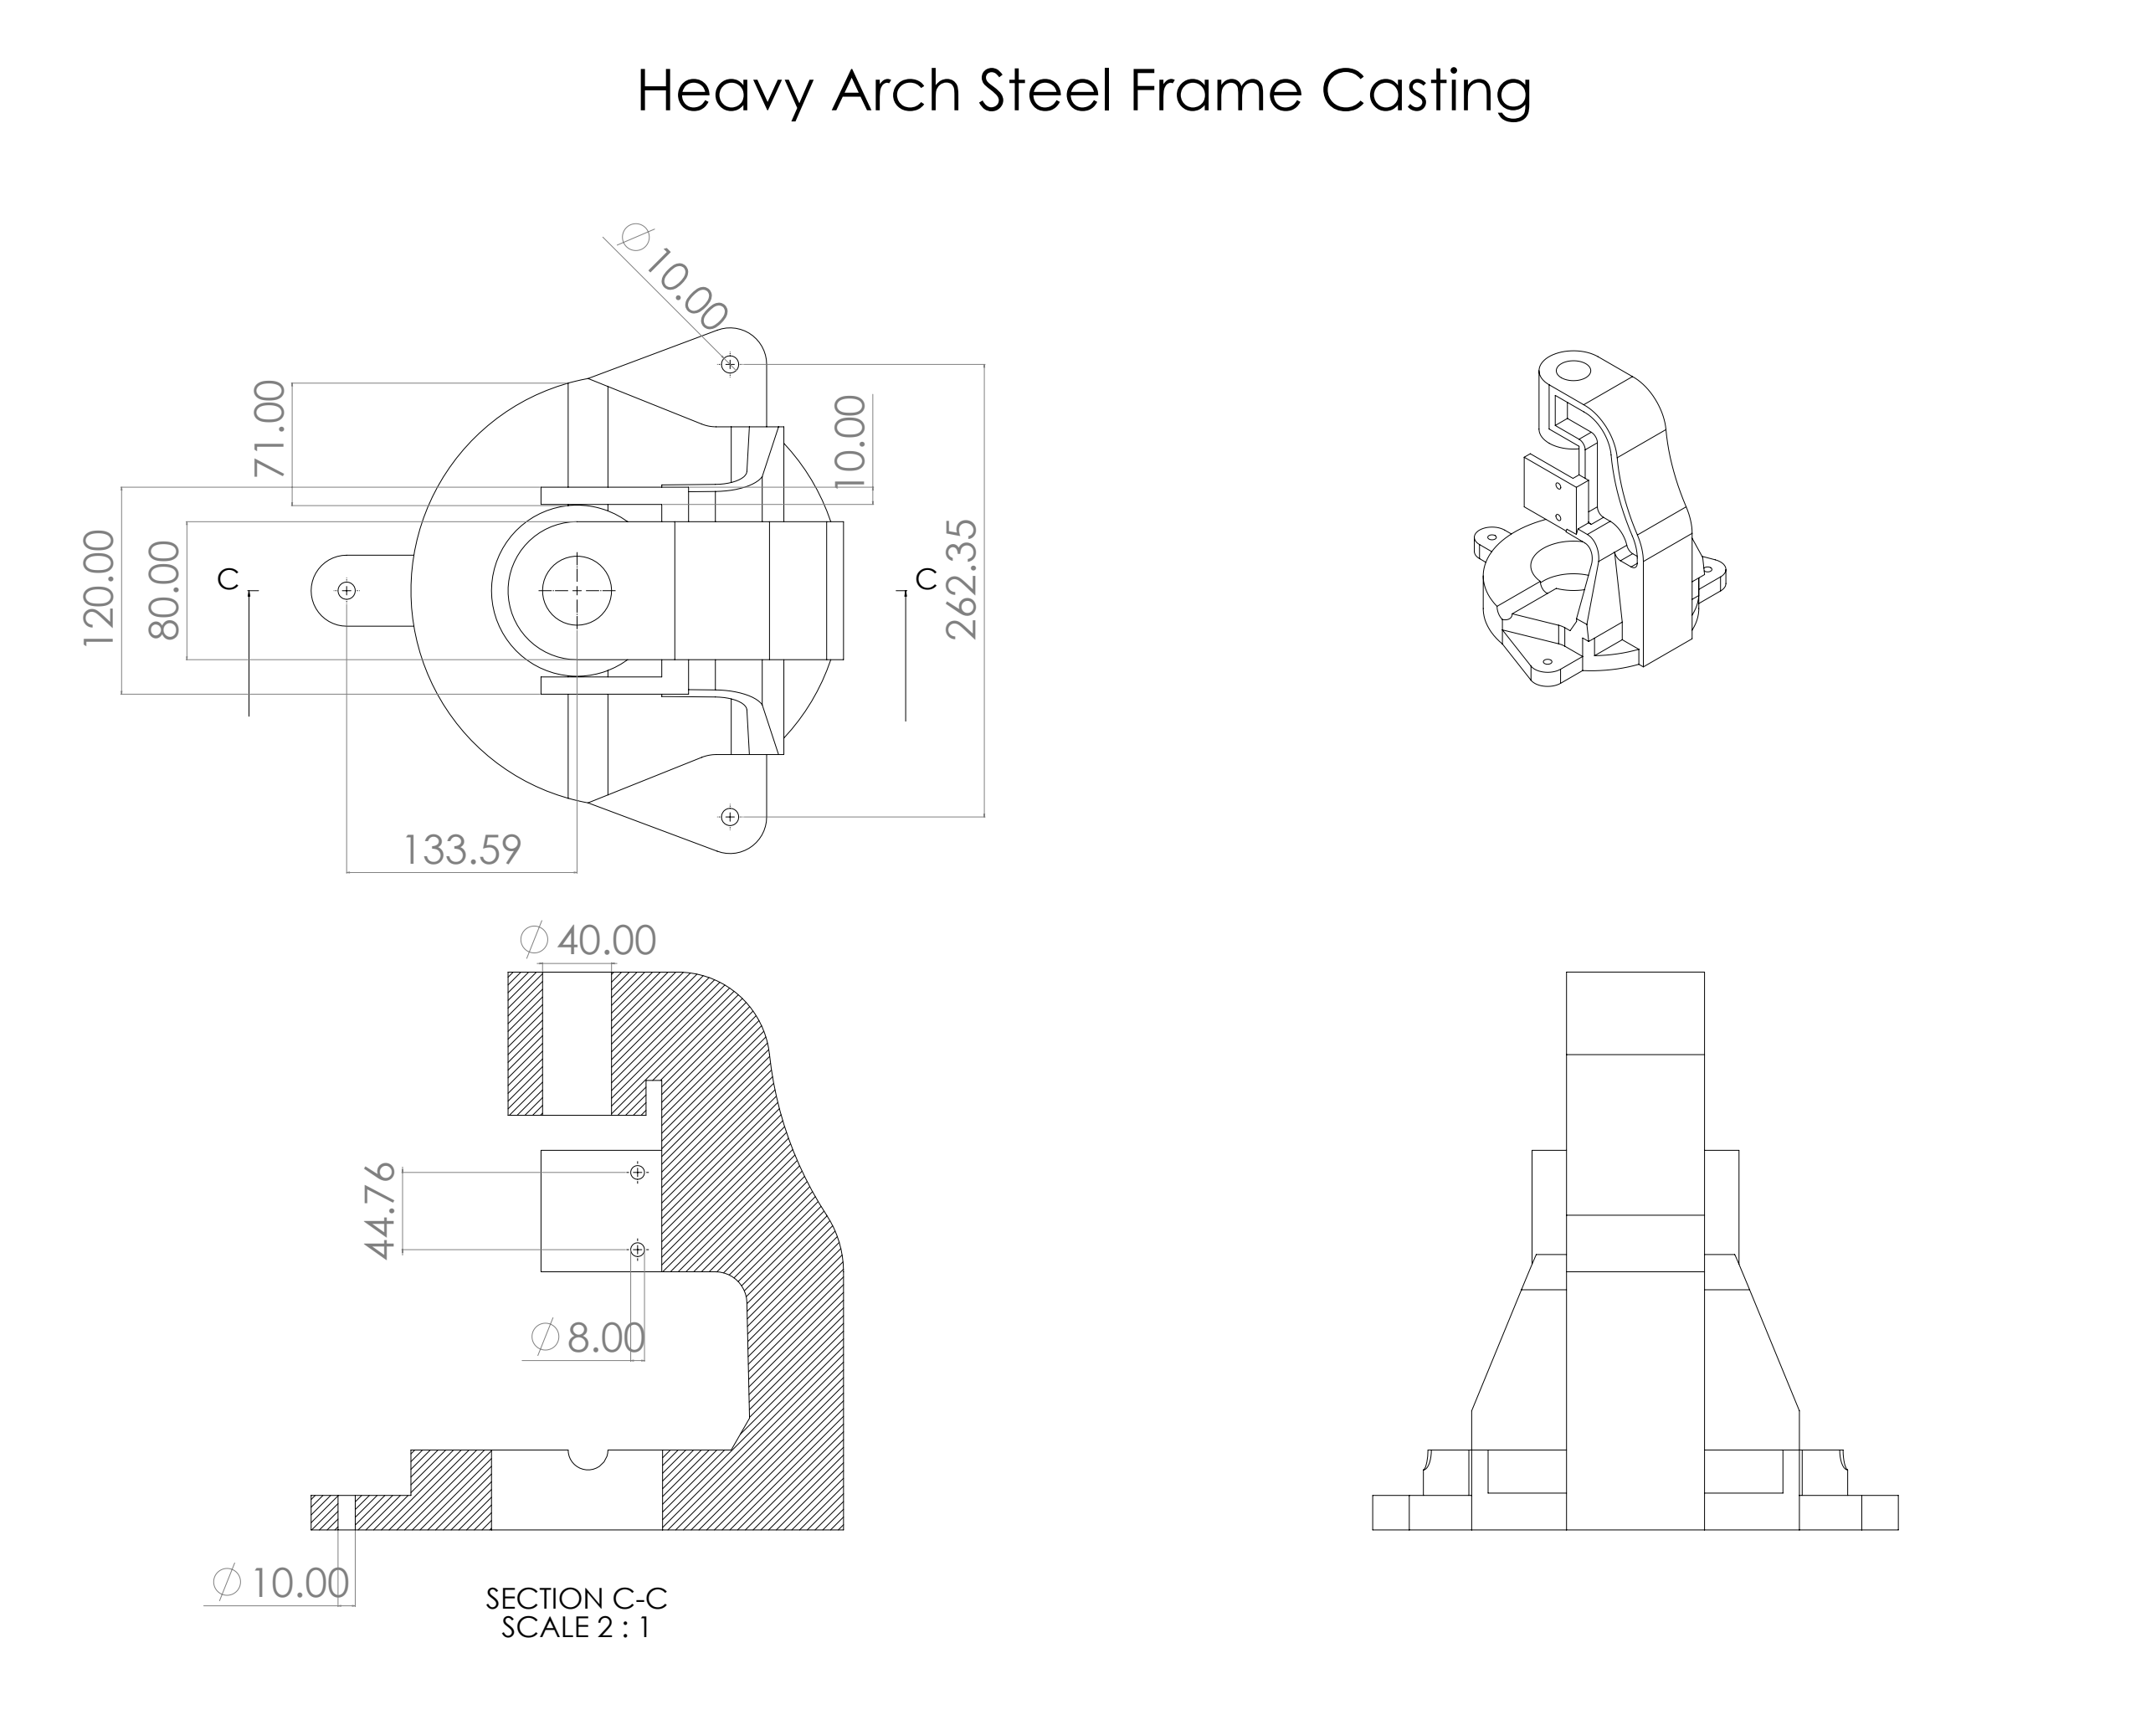
ISO-10303-21;
HEADER;
FILE_DESCRIPTION (('STEP AP214'),
    '1' );
FILE_NAME ('Heavy Arch Steel Frame Casting.step',
    '2026-10-24T00:28:05',
    ( '' ),
    ( '' ),
    'SwSTEP 2.0',
    'SolidWorks 2025',
    '' );
FILE_SCHEMA (( 'AUTOMOTIVE_DESIGN' ));
ENDSEC;

DATA;
#3=VECTOR ( 'NONE', #11444, 1000.000000000000000 ) ;
#4=DIRECTION ( 'NONE',  ( 0.000000000000000000, -1.000000000000000000, 0.000000000000000000 ) ) ;
#8=DIRECTION ( 'NONE',  ( -0.000000000000000000, -0.000000000000000000, -1.000000000000000000 ) ) ;
#9=ORIENTED_EDGE ( 'NONE', *, *, #63, .F. ) ;
#13=VERTEX_POINT ( 'NONE', #14894 ) ;
#23=CARTESIAN_POINT ( 'NONE',  ( 20.42502041961814641, 160.1716627696692683, -50.00000000000000000 ) ) ;
#25=DIRECTION ( 'NONE',  ( 0.000000000000000000, 0.000000000000000000, 1.000000000000000000 ) ) ;
#26=AXIS2_PLACEMENT_3D ( 'NONE', #1810, #8485, #15108 ) ;
#28=CARTESIAN_POINT ( 'NONE',  ( -33.09803238365465461, 52.74628974220605215, 120.5385558893279807 ) ) ;
#30=CARTESIAN_POINT ( 'NONE',  ( -10.76731745429009912, 56.85652257517428865, 118.3724535612433186 ) ) ;
#32=( GEOMETRIC_REPRESENTATION_CONTEXT ( 3 ) GLOBAL_UNCERTAINTY_ASSIGNED_CONTEXT ( ( #4204 ) ) GLOBAL_UNIT_ASSIGNED_CONTEXT ( ( #10723, #14002, #17024 ) ) REPRESENTATION_CONTEXT ( 'NONE', 'WORKASPACE' ) );
#35=ORIENTED_EDGE ( 'NONE', *, *, #14468, .F. ) ;
#40=AXIS2_PLACEMENT_3D ( 'NONE', #19318, #13155, #16192 ) ;
#59=CARTESIAN_POINT ( 'NONE',  ( 115.7989814974898337, 152.5259582928263740, 40.00000000000000000 ) ) ;
#60=DIRECTION ( 'NONE',  ( 1.000000000000000000, 9.855701800883827197E-17, 0.000000000000000000 ) ) ;
#63=EDGE_CURVE ( 'NONE', #14197, #16401, #15913, .T. ) ;
#68=CARTESIAN_POINT ( 'NONE',  ( -22.30770786884145451, -343.0245277843623057, -122.9933582338429687 ) ) ;
#70=CARTESIAN_POINT ( 'NONE',  ( 20.42502041961814641, 160.1716627696692683, 49.99999999999999289 ) ) ;
#73=ADVANCED_FACE ( 'NONE', ( #292 ), #3940, .T. ) ;
#85=CARTESIAN_POINT ( 'NONE',  ( -11.33174043645153262, 53.25345476394927857, -46.46619372074344767 ) ) ;
#89=FACE_OUTER_BOUND ( 'NONE', #5371, .T. ) ;
#91=DIRECTION ( 'NONE',  ( 1.854788578061058554E-16, 1.000000000000000000, 0.000000000000000000 ) ) ;
#94=CARTESIAN_POINT ( 'NONE',  ( -10.76731745429010090, 56.85652257517428865, -152.3753892284480003 ) ) ;
#96=DIRECTION ( 'NONE',  ( -1.000000000000000000, 0.000000000000000000, 0.000000000000000000 ) ) ;
#100=CARTESIAN_POINT ( 'NONE',  ( -28.68588794268872277, 230.8848358243226073, -40.00000000000000000 ) ) ;
#105=ORIENTED_EDGE ( 'NONE', *, *, #199, .F. ) ;
#107=EDGE_CURVE ( 'NONE', #16081, #2296, #14541, .T. ) ;
#113=EDGE_CURVE ( 'NONE', #8154, #14441, #20281, .T. ) ;
#116=CARTESIAN_POINT ( 'NONE',  ( 69.79185940953689737, 142.2976266388001250, 69.11456258820065557 ) ) ;
#117=AXIS2_PLACEMENT_3D ( 'NONE', #15282, #17003, #20238 ) ;
#123=ORIENTED_EDGE ( 'NONE', *, *, #2940, .T. ) ;
#132=ORIENTED_EDGE ( 'NONE', *, *, #11871, .F. ) ;
#146=CARTESIAN_POINT ( 'NONE',  ( 20.42502041961814641, 160.1716627696692683, 61.32762281133329196 ) ) ;
#150=VECTOR ( 'NONE', #6440, 1000.000000000000000 ) ;
#154=VECTOR ( 'NONE', #10153, 1000.000000000000000 ) ;
#155=ORIENTED_EDGE ( 'NONE', *, *, #15237, .F. ) ;
#157=EDGE_LOOP ( 'NONE', ( #5136, #14998, #4320, #2465 ) ) ;
#168=DIRECTION ( 'NONE',  ( 0.000000000000000000, 0.000000000000000000, -1.000000000000000000 ) ) ;
#174=LINE ( 'NONE', #10093, #7830 ) ;
#179=EDGE_CURVE ( 'NONE', #20702, #11681, #8806, .T. ) ;
#182=VERTEX_POINT ( 'NONE', #608 ) ;
#184=ORIENTED_EDGE ( 'NONE', *, *, #5125, .F. ) ;
#188=ORIENTED_EDGE ( 'NONE', *, *, #12536, .T. ) ;
#193=CARTESIAN_POINT ( 'NONE',  ( -18.46114582419561856, 45.97303840584705625, -48.53623208051946136 ) ) ;
#195=CARTESIAN_POINT ( 'NONE',  ( 71.32175588950862277, 75.31183677523708297, 40.00000000000000000 ) ) ;
#199=EDGE_CURVE ( 'NONE', #182, #19453, #6902, .T. ) ;
#206=CARTESIAN_POINT ( 'NONE',  ( -31.47597222270714212, 49.78415940255306538, -49.52648848774079937 ) ) ;
#216=ORIENTED_EDGE ( 'NONE', *, *, #18810, .T. ) ;
#219=EDGE_CURVE ( 'NONE', #12803, #14751, #2645, .T. ) ;
#227=CARTESIAN_POINT ( 'NONE',  ( 60.03793209889851568, 30.52886280891152282, -131.1729372809869005 ) ) ;
#230=ORIENTED_EDGE ( 'NONE', *, *, #2551, .F. ) ;
#234=ORIENTED_EDGE ( 'NONE', *, *, #8898, .F. ) ;
#243=VECTOR ( 'NONE', #20484, 1000.000000000000000 ) ;
#245=DIRECTION ( 'NONE',  ( -1.000000000000000000, 0.000000000000000000, 0.000000000000000000 ) ) ;
#258=VERTEX_POINT ( 'NONE', #20385 ) ;
#264=VERTEX_POINT ( 'NONE', #824 ) ;
#281=CARTESIAN_POINT ( 'NONE',  ( 79.78925230247502043, 142.5259582928263455, -20.00000000000000355 ) ) ;
#292=FACE_OUTER_BOUND ( 'NONE', #157, .T. ) ;
#297=CARTESIAN_POINT ( 'NONE',  ( -13.97728958318061565, 48.85369832438319548, -47.37148056848186428 ) ) ;
#299=DIRECTION ( 'NONE',  ( 1.000000000000000000, 0.000000000000000000, 0.000000000000000000 ) ) ;
#300=EDGE_CURVE ( 'NONE', #14946, #18462, #14017, .T. ) ;
#305=DIRECTION ( 'NONE',  ( 0.000000000000000000, 1.000000000000000000, 0.000000000000000000 ) ) ;
#310=CARTESIAN_POINT ( 'NONE',  ( -28.68588794268872988, 47.23886018424757083, -49.60091809715359545 ) ) ;
#317=ORIENTED_EDGE ( 'NONE', *, *, #11658, .T. ) ;
#323=AXIS2_PLACEMENT_3D ( 'NONE', #6998, #18893, #7103 ) ;
#352=VECTOR ( 'NONE', #18176, 1000.000000000000000 ) ;
#359=CARTESIAN_POINT ( 'NONE',  ( 0.000000000000000000, 56.85652257517428865, 0.000000000000000000 ) ) ;
#376=VECTOR ( 'NONE', #7717, 1000.000000000000000 ) ;
#385=CARTESIAN_POINT ( 'NONE',  ( 30.42502041961813575, 271.1055109169419097, 20.00000000000000355 ) ) ;
#387=CARTESIAN_POINT ( 'NONE',  ( 81.24038404635966515, 10.52886280891152104, -94.99999999999994316 ) ) ;
#389=ADVANCED_FACE ( 'NONE', ( #7915 ), #13016, .F. ) ;
#392=CIRCLE ( 'NONE', #11415, 9.999999999999994671 ) ;
#393=CARTESIAN_POINT ( 'NONE',  ( 81.24038404635966515, 10.52886280891152104, 94.99999999999994316 ) ) ;
#396=ORIENTED_EDGE ( 'NONE', *, *, #3873, .T. ) ;
#399=VECTOR ( 'NONE', #1589, 1000.000000000000000 ) ;
#402=EDGE_LOOP ( 'NONE', ( #20811, #2569, #4602, #6698 ) ) ;
#407=CARTESIAN_POINT ( 'NONE',  ( -28.68588794268872988, 47.23886018424757083, -49.60091809715359545 ) ) ;
#411=DIRECTION ( 'NONE',  ( 0.000000000000000000, -1.000000000000000000, 0.000000000000000000 ) ) ;
#426=ORIENTED_EDGE ( 'NONE', *, *, #17683, .T. ) ;
#428=CARTESIAN_POINT ( 'NONE',  ( 30.07572094023280940, 170.1716627696692683, -57.31989048965873934 ) ) ;
#430=ORIENTED_EDGE ( 'NONE', *, *, #1923, .F. ) ;
#431=FACE_OUTER_BOUND ( 'NONE', #16031, .T. ) ;
#440=EDGE_CURVE ( 'NONE', #16030, #15607, #16966, .T. ) ;
#443=ORIENTED_EDGE ( 'NONE', *, *, #8517, .T. ) ;
#446=ORIENTED_EDGE ( 'NONE', *, *, #9956, .F. ) ;
#450=AXIS2_PLACEMENT_3D ( 'NONE', #15921, #17640, #8987 ) ;
#451=VERTEX_POINT ( 'NONE', #3287 ) ;
#454=VERTEX_POINT ( 'NONE', #16805 ) ;
#464=CARTESIAN_POINT ( 'NONE',  ( -26.01014438536011397, 45.91972051657856468, 122.2644972899424687 ) ) ;
#466=LINE ( 'NONE', #566, #15334 ) ;
#475=ORIENTED_EDGE ( 'NONE', *, *, #15442, .F. ) ;
#493=AXIS2_PLACEMENT_3D ( 'NONE', #1831, #8402, #15027 ) ;
#494=CARTESIAN_POINT ( 'NONE',  ( 81.24038404635965094, 10.52886280891152104, -131.1729372809869005 ) ) ;
#496=AXIS2_PLACEMENT_3D ( 'NONE', #18707, #14078, #15484 ) ;
#504=EDGE_LOOP ( 'NONE', ( #18852, #5687, #1345, #9828 ) ) ;
#509=ORIENTED_EDGE ( 'NONE', *, *, #7343, .F. ) ;
#514=CARTESIAN_POINT ( 'NONE',  ( 52.60622592008805043, 30.52886280891152282, -151.0302712373927250 ) ) ;
#525=DIRECTION ( 'NONE',  ( -0.000000000000000000, -0.000000000000000000, -1.000000000000000000 ) ) ;
#527=ORIENTED_EDGE ( 'NONE', *, *, #5440, .F. ) ;
#534=VERTEX_POINT ( 'NONE', #5742 ) ;
#549=ORIENTED_EDGE ( 'NONE', *, *, #4990, .T. ) ;
#554=VERTEX_POINT ( 'NONE', #14098 ) ;
#566=CARTESIAN_POINT ( 'NONE',  ( -74.06037022053952512, 10.52886280891152104, -40.00000000000000000 ) ) ;
#572=EDGE_LOOP ( 'NONE', ( #20946, #19765, #20650 ) ) ;
#588=CARTESIAN_POINT ( 'NONE',  ( 35.96497763894178945, 230.5765313837437418, -40.00000000000000000 ) ) ;
#592=DIRECTION ( 'NONE',  ( -0.000000000000000000, -0.000000000000000000, -1.000000000000000000 ) ) ;
#595=EDGE_CURVE ( 'NONE', #1881, #15561, #10610, .T. ) ;
#596=CIRCLE ( 'NONE', #11637, 4.000000000000003553 ) ;
#602=ORIENTED_EDGE ( 'NONE', *, *, #17756, .T. ) ;
#604=VERTEX_POINT ( 'NONE', #20679 ) ;
#606=LINE ( 'NONE', #100, #18425 ) ;
#607=EDGE_CURVE ( 'NONE', #10104, #12829, #18832, .T. ) ;
#608=CARTESIAN_POINT ( 'NONE',  ( -28.68588794268874054, 271.1055109169419666, 40.00000000000000000 ) ) ;
#610=ORIENTED_EDGE ( 'NONE', *, *, #4427, .T. ) ;
#615=LINE ( 'NONE', #17154, #5483 ) ;
#632=ORIENTED_EDGE ( 'NONE', *, *, #5260, .T. ) ;
#639=CARTESIAN_POINT ( 'NONE',  ( -28.68588794268873698, 10.52886280891152104, 0.000000000000000000 ) ) ;
#647=CARTESIAN_POINT ( 'NONE',  ( 60.03793209889851568, 30.52886280891152282, 131.1729372809869005 ) ) ;
#649=ADVANCED_FACE ( 'NONE', ( #4241 ), #12780, .T. ) ;
#651=DIRECTION ( 'NONE',  ( -0.000000000000000000, -0.000000000000000000, 1.000000000000000000 ) ) ;
#653=CIRCLE ( 'NONE', #14480, 21.20245194746113526 ) ;
#671=AXIS2_PLACEMENT_3D ( 'NONE', #5649, #6070, #7583 ) ;
#680=EDGE_LOOP ( 'NONE', ( #16620, #509, #5345, #8208 ) ) ;
#684=CARTESIAN_POINT ( 'NONE',  ( 115.7989814974898337, 152.5259582928263740, -20.00000000000000355 ) ) ;
#696=DIRECTION ( 'NONE',  ( 1.000000000000000000, 0.000000000000000000, 0.000000000000000000 ) ) ;
#698=FACE_OUTER_BOUND ( 'NONE', #4314, .T. ) ;
#700=DIRECTION ( 'NONE',  ( -0.000000000000000000, -0.000000000000000000, -1.000000000000000000 ) ) ;
#703=DIRECTION ( 'NONE',  ( 0.000000000000000000, -1.000000000000000000, 0.000000000000000000 ) ) ;
#706=ORIENTED_EDGE ( 'NONE', *, *, #13101, .F. ) ;
#714=ORIENTED_EDGE ( 'NONE', *, *, #20644, .F. ) ;
#717=EDGE_CURVE ( 'NONE', #20672, #5108, #13166, .T. ) ;
#723=DIRECTION ( 'NONE',  ( 0.000000000000000000, -0.000000000000000000, -1.000000000000000000 ) ) ;
#727=FACE_OUTER_BOUND ( 'NONE', #18825, .T. ) ;
#728=CLOSED_SHELL ( 'NONE', ( #4202, #18729, #7183, #1313, #6098, #14803, #2877, #2308, #8698, #9259, #1514, #21123, #2681, #8425, #4950, #3532, #389, #2715, #19260, #14653, #15130, #14125, #19463, #13734, #19883, #19785, #7149, #16387, #12129, #10656, #9205, #12272, #16233, #3470, #2143, #15969, #3158, #11966, #8090, #20749, #11190, #649, #18699, #8016, #5574, #907, #20543, #1966, #6567, #13747, #21117, #1097, #12190, #73, #11691, #16866, #10538, #19874, #8200, #12587, #9693, #14131, #2231, #11601, #7880, #15316, #13856, #1907, #10138, #3997, #11879, #20146, #15364, #1047, #17279, #12993, #4417, #13206, #9791, #6710, #19859, #8106, #17682, #4283, #12076, #13479, #20733, #20323, #20863, #3939, #1701, #7829, #2906, #15283, #6218, #20450, #19796, #1639, #4404, #10989, #20740, #14224, #2354, #839, #7752, #14892, #15777, #1840, #3193, #15792, #9164, #1436, #7801, #12477, #8633, #18193, #14455, #9085, #11057 ) ) ;
#730=EDGE_CURVE ( 'NONE', #15685, #3984, #3339, .T. ) ;
#739=VERTEX_POINT ( 'NONE', #17751 ) ;
#754=CARTESIAN_POINT ( 'NONE',  ( 52.94681837068318941, 78.74778544605769071, -94.99999999999994316 ) ) ;
#763=VERTEX_POINT ( 'NONE', #10929 ) ;
#764=CARTESIAN_POINT ( 'NONE',  ( 292.4526463419396691, 308.2087638784415162, 20.00000000000000355 ) ) ;
#765=ORIENTED_EDGE ( 'NONE', *, *, #15458, .T. ) ;
#772=ORIENTED_EDGE ( 'NONE', *, *, #7755, .F. ) ;
#779=DIRECTION ( 'NONE',  ( 0.000000000000000000, -1.000000000000000000, 0.000000000000000000 ) ) ;
#785=PRODUCT_DEFINITION_CONTEXT ( 'detailed design', #9294, 'design' ) ;
#790=AXIS2_PLACEMENT_3D ( 'NONE', #4343, #10924, #17535 ) ;
#793=ORIENTED_EDGE ( 'NONE', *, *, #1569, .T. ) ;
#795=VERTEX_POINT ( 'NONE', #9310 ) ;
#796=LINE ( 'NONE', #2405, #6289 ) ;
#806=DIRECTION ( 'NONE',  ( -0.000000000000000000, -0.000000000000000000, 1.000000000000000000 ) ) ;
#808=CARTESIAN_POINT ( 'NONE',  ( 0.000000000000000000, 0.000000000000000000, 0.000000000000000000 ) ) ;
#814=CARTESIAN_POINT ( 'NONE',  ( -33.24036626417445461, 53.08430543508956134, -120.4996691248974656 ) ) ;
#824=CARTESIAN_POINT ( 'NONE',  ( -49.57497958038186425, 230.5765313837437418, 60.00000000000000000 ) ) ;
#834=DIRECTION ( 'NONE',  ( 1.000000000000000000, 0.000000000000000000, 0.000000000000000000 ) ) ;
#835=CARTESIAN_POINT ( 'NONE',  ( 6.416697501590670427, 172.9933428177121471, -60.00000000000000000 ) ) ;
#836=CIRCLE ( 'NONE', #10824, 21.20245194746113526 ) ;
#839=ADVANCED_FACE ( 'NONE', ( #6238 ), #6566, .T. ) ;
#840=CARTESIAN_POINT ( 'NONE',  ( 6.416697501590670427, 217.7548513357008630, 49.99999999999999289 ) ) ;
#847=ORIENTED_EDGE ( 'NONE', *, *, #2670, .F. ) ;
#851=CARTESIAN_POINT ( 'NONE',  ( 105.7989814974898479, 152.5259582928263740, 20.00000000000000355 ) ) ;
#857=FACE_OUTER_BOUND ( 'NONE', #9920, .T. ) ;
#858=CARTESIAN_POINT ( 'NONE',  ( -28.68588794268872277, 174.3162933293988033, -20.00000000000000000 ) ) ;
#861=DIRECTION ( 'NONE',  ( 0.000000000000000000, -1.000000000000000000, 0.000000000000000000 ) ) ;
#865=DIRECTION ( 'NONE',  ( -0.000000000000000000, -0.000000000000000000, -1.000000000000000000 ) ) ;
#871=ORIENTED_EDGE ( 'NONE', *, *, #21201, .F. ) ;
#874=EDGE_LOOP ( 'NONE', ( #5710, #13740, #20222, #9194 ) ) ;
#880=VERTEX_POINT ( 'NONE', #1839 ) ;
#889=LINE ( 'NONE', #9296, #7146 ) ;
#895=ORIENTED_EDGE ( 'NONE', *, *, #3138, .F. ) ;
#898=ORIENTED_EDGE ( 'NONE', *, *, #6988, .F. ) ;
#907=ADVANCED_FACE ( 'NONE', ( #11663 ), #10238, .F. ) ;
#912=DIRECTION ( 'NONE',  ( -0.02112707654195870172, 0.9250389998264586522, -0.3792841882241536067 ) ) ;
#928=DIRECTION ( 'NONE',  ( 0.000000000000000000, -1.000000000000000000, 0.000000000000000000 ) ) ;
#931=CYLINDRICAL_SURFACE ( 'NONE', #21088, 125.0000000000000000 ) ;
#939=CARTESIAN_POINT ( 'NONE',  ( 79.78925230247502043, 142.5259582928263455, -40.00000000000000000 ) ) ;
#940=CARTESIAN_POINT ( 'NONE',  ( 20.42502041961813930, 230.5765313837437418, 60.00000000000000000 ) ) ;
#947=VECTOR ( 'NONE', #1680, 1000.000000000000114 ) ;
#948=DIRECTION ( 'NONE',  ( 0.000000000000000000, -1.000000000000000000, 0.000000000000000000 ) ) ;
#950=DIRECTION ( 'NONE',  ( 0.000000000000000000, -1.000000000000000000, 0.000000000000000000 ) ) ;
#952=VERTEX_POINT ( 'NONE', #10343 ) ;
#954=ORIENTED_EDGE ( 'NONE', *, *, #14883, .F. ) ;
#956=AXIS2_PLACEMENT_3D ( 'NONE', #2213, #8797, #5337 ) ;
#961=EDGE_LOOP ( 'NONE', ( #6161, #9124, #13988, #14252 ) ) ;
#970=DIRECTION ( 'NONE',  ( 0.000000000000000000, -1.000000000000000000, 0.000000000000000000 ) ) ;
#973=AXIS2_PLACEMENT_3D ( 'NONE', #2028, #2337, #11954 ) ;
#983=VERTEX_POINT ( 'NONE', #16655 ) ;
#989=ORIENTED_EDGE ( 'NONE', *, *, #1574, .T. ) ;
#997=CARTESIAN_POINT ( 'NONE',  ( 28.16023193154655502, 323.8848358243226357, 40.00000000000000000 ) ) ;
#998=DIRECTION ( 'NONE',  ( -1.374938938973709817E-16, 1.000000000000000000, 0.000000000000000000 ) ) ;
#1002=VERTEX_POINT ( 'NONE', #8832 ) ;
#1007=ORIENTED_EDGE ( 'NONE', *, *, #9742, .T. ) ;
#1017=AXIS2_PLACEMENT_3D ( 'NONE', #12084, #13620, #8731 ) ;
#1019=DIRECTION ( 'NONE',  ( 1.000000000000000000, 0.000000000000000000, 0.000000000000000000 ) ) ;
#1022=CARTESIAN_POINT ( 'NONE',  ( -18.68588794268873698, 323.8848358243226357, -40.00000000000000000 ) ) ;
#1030=ORIENTED_EDGE ( 'NONE', *, *, #13546, .T. ) ;
#1032=EDGE_LOOP ( 'NONE', ( #18693, #12072, #7439, #4372, #20196, #8855, #4075 ) ) ;
#1033=CARTESIAN_POINT ( 'NONE',  ( 115.7989814974898337, 142.5259582928263455, 20.00000000000000355 ) ) ;
#1038=ORIENTED_EDGE ( 'NONE', *, *, #21391, .T. ) ;
#1040=CARTESIAN_POINT ( 'NONE',  ( 72.94945500224395118, 285.0140030772282103, -20.00000000000000355 ) ) ;
#1046=PLANE ( 'NONE',  #18730 ) ;
#1047=ADVANCED_FACE ( 'NONE', ( #431 ), #16968, .F. ) ;
#1049=CIRCLE ( 'NONE', #11375, 210.7252770684331438 ) ;
#1051=CARTESIAN_POINT ( 'NONE',  ( 51.93385628276429600, 30.52886280891152282, 94.99999999999994316 ) ) ;
#1055=CARTESIAN_POINT ( 'NONE',  ( 78.68120802659203150, 149.7457237375499517, 40.00000000000000000 ) ) ;
#1066=ORIENTED_EDGE ( 'NONE', *, *, #6841, .F. ) ;
#1075=LINE ( 'NONE', #12307, #15304 ) ;
#1078=CARTESIAN_POINT ( 'NONE',  ( 35.96497763894178945, 230.5765313837437418, -40.00000000000000000 ) ) ;
#1082=CIRCLE ( 'NONE', #2490, 4.000000000000003553 ) ;
#1084=VECTOR ( 'NONE', #12802, 1000.000000000000000 ) ;
#1097=ADVANCED_FACE ( 'NONE', ( #10662 ), #9263, .T. ) ;
#1121=EDGE_CURVE ( 'NONE', #8313, #3421, #9046, .T. ) ;
#1126=LINE ( 'NONE', #9431, #4731 ) ;
#1127=CARTESIAN_POINT ( 'NONE',  ( -49.57497958038185715, 160.1716627696692683, 60.00000000000000000 ) ) ;
#1128=DIRECTION ( 'NONE',  ( -0.9365583756827543516, 0.000000000000000000, -0.3505116388060184329 ) ) ;
#1129=VECTOR ( 'NONE', #91, 1000.000000000000000 ) ;
#1136=LINE ( 'NONE', #6295, #19374 ) ;
#1137=EDGE_LOOP ( 'NONE', ( #13123, #13935, #1985, #5078, #11029, #2986, #11526, #5417, #8051, #16113 ) ) ;
#1138=DIRECTION ( 'NONE',  ( 0.000000000000000000, 0.000000000000000000, -1.000000000000000000 ) ) ;
#1141=DIRECTION ( 'NONE',  ( 0.000000000000000000, 0.000000000000000000, 1.000000000000000000 ) ) ;
#1143=EDGE_LOOP ( 'NONE', ( #7066, #7328 ) ) ;
#1149=CARTESIAN_POINT ( 'NONE',  ( 0.000000000000000000, 56.85652257517428865, 0.000000000000000000 ) ) ;
#1150=DIRECTION ( 'NONE',  ( 0.000000000000000000, 0.000000000000000000, 1.000000000000000000 ) ) ;
#1151=FACE_OUTER_BOUND ( 'NONE', #4117, .T. ) ;
#1152=CARTESIAN_POINT ( 'NONE',  ( 60.03793209889851568, 10.52886280891152104, 131.1729372809869005 ) ) ;
#1155=VECTOR ( 'NONE', #14617, 1000.000000000000114 ) ;
#1161=VERTEX_POINT ( 'NONE', #5802 ) ;
#1165=VERTEX_POINT ( 'NONE', #17487 ) ;
#1171=DIRECTION ( 'NONE',  ( 0.000000000000000000, 0.000000000000000000, 1.000000000000000000 ) ) ;
#1175=CARTESIAN_POINT ( 'NONE',  ( 30.42502041961813575, 271.1055109169419097, -40.00000000000000000 ) ) ;
#1186=VECTOR ( 'NONE', #651, 1000.000000000000000 ) ;
#1199=VECTOR ( 'NONE', #3391, 1000.000000000000000 ) ;
#1205=LINE ( 'NONE', #17735, #6578 ) ;
#1206=CARTESIAN_POINT ( 'NONE',  ( -18.68588794268873698, 323.8848358243226357, 20.00000000000000355 ) ) ;
#1209=ORIENTED_EDGE ( 'NONE', *, *, #18529, .T. ) ;
#1211=ORIENTED_EDGE ( 'NONE', *, *, #11510, .F. ) ;
#1214=DIRECTION ( 'NONE',  ( 0.000000000000000000, 1.000000000000000000, 0.000000000000000000 ) ) ;
#1218=CARTESIAN_POINT ( 'NONE',  ( 51.50493485826542184, 141.8799693780962912, 20.00000000000000355 ) ) ;
#1229=DIRECTION ( 'NONE',  ( 0.008660258604321402487, -0.3791853047755957551, 0.9252802302887190855 ) ) ;
#1234=EDGE_CURVE ( 'NONE', #182, #5454, #6020, .T. ) ;
#1242=ORIENTED_EDGE ( 'NONE', *, *, #14883, .T. ) ;
#1244=FACE_OUTER_BOUND ( 'NONE', #10818, .T. ) ;
#1256=EDGE_CURVE ( 'NONE', #17485, #13185, #15990, .T. ) ;
#1259=DIRECTION ( 'NONE',  ( 0.000000000000000000, 0.000000000000000000, -1.000000000000000000 ) ) ;
#1268=CARTESIAN_POINT ( 'NONE',  ( 10.41669750159067220, 172.9933428177121471, -50.00000000000000000 ) ) ;
#1270=CYLINDRICAL_SURFACE ( 'NONE', #7188, 10.00000000000000355 ) ;
#1271=DIRECTION ( 'NONE',  ( -0.000000000000000000, -0.000000000000000000, 1.000000000000000000 ) ) ;
#1275=LINE ( 'NONE', #14482, #18370 ) ;
#1286=AXIS2_PLACEMENT_3D ( 'NONE', #15307, #20265, #17237 ) ;
#1295=EDGE_CURVE ( 'NONE', #6060, #10209, #5912, .T. ) ;
#1296=CIRCLE ( 'NONE', #17189, 40.00000000000000000 ) ;
#1303=EDGE_CURVE ( 'NONE', #4099, #4231, #20951, .T. ) ;
#1310=CARTESIAN_POINT ( 'NONE',  ( 51.50493485826542184, 141.8799693780962912, 40.00000000000000000 ) ) ;
#1313=ADVANCED_FACE ( 'NONE', ( #14577 ), #8057, .T. ) ;
#1316=VERTEX_POINT ( 'NONE', #9580 ) ;
#1323=CARTESIAN_POINT ( 'NONE',  ( -162.2727221670389781, 30.52886280891152282, 0.000000000000000000 ) ) ;
#1336=EDGE_LOOP ( 'NONE', ( #2701, #4093, #17098, #4444 ) ) ;
#1339=LINE ( 'NONE', #4681, #4640 ) ;
#1340=CIRCLE ( 'NONE', #13434, 5.000000000000004441 ) ;
#1345=ORIENTED_EDGE ( 'NONE', *, *, #1971, .T. ) ;
#1348=CARTESIAN_POINT ( 'NONE',  ( 88.28695088269886071, 152.5259582928263740, -20.00000000000000355 ) ) ;
#1351=DIRECTION ( 'NONE',  ( 0.000000000000000000, 0.000000000000000000, 1.000000000000000000 ) ) ;
#1355=EDGE_CURVE ( 'NONE', #18698, #18459, #11098, .T. ) ;
#1356=CARTESIAN_POINT ( 'NONE',  ( 91.21585410611801592, 56.85652257517428865, 94.99999999999994316 ) ) ;
#1365=ORIENTED_EDGE ( 'NONE', *, *, #5370, .T. ) ;
#1375=DIRECTION ( 'NONE',  ( -1.000000000000000000, 0.000000000000000000, -2.399110633850889130E-16 ) ) ;
#1379=CARTESIAN_POINT ( 'NONE',  ( 40.42502041961814996, 170.1716627696692683, -20.00000000000000355 ) ) ;
#1381=CARTESIAN_POINT ( 'NONE',  ( -28.68588794268874054, 333.8848358243226357, 40.00000000000000000 ) ) ;
#1382=EDGE_CURVE ( 'NONE', #14089, #19571, #18016, .T. ) ;
#1392=EDGE_CURVE ( 'NONE', #1858, #4099, #16411, .T. ) ;
#1394=EDGE_LOOP ( 'NONE', ( #2018, #1886, #15579, #4337 ) ) ;
#1396=DIRECTION ( 'NONE',  ( 0.000000000000000000, 1.000000000000000000, 0.000000000000000000 ) ) ;
#1399=CIRCLE ( 'NONE', #13495, 21.20245194746113526 ) ;
#1404=DIRECTION ( 'NONE',  ( 0.000000000000000000, 0.000000000000000000, -1.000000000000000000 ) ) ;
#1413=CARTESIAN_POINT ( 'NONE',  ( -49.57497958038185715, 160.1716627696692683, -50.00000000000000000 ) ) ;
#1414=EDGE_LOOP ( 'NONE', ( #2541, #10703, #17353, #15763, #10706 ) ) ;
#1422=EDGE_CURVE ( 'NONE', #18669, #17480, #19322, .T. ) ;
#1436=ADVANCED_FACE ( 'NONE', ( #4509 ), #9895, .T. ) ;
#1442=CIRCLE ( 'NONE', #11790, 28.29169339157297358 ) ;
#1445=ORIENTED_EDGE ( 'NONE', *, *, #3274, .F. ) ;
#1446=DIRECTION ( 'NONE',  ( -0.000000000000000000, 1.000000000000000000, -0.000000000000000000 ) ) ;
#1447=VERTEX_POINT ( 'NONE', #1268 ) ;
#1457=CARTESIAN_POINT ( 'NONE',  ( -28.68588794268873343, 47.23886018424757083, 49.60091809715359545 ) ) ;
#1474=ORIENTED_EDGE ( 'NONE', *, *, #8471, .T. ) ;
#1480=DIRECTION ( 'NONE',  ( 1.000000000000000000, 0.000000000000000000, -0.000000000000000000 ) ) ;
#1483=EDGE_CURVE ( 'NONE', #1002, #15603, #7743, .T. ) ;
#1485=DIRECTION ( 'NONE',  ( -1.232945044042657126E-32, 9.855701800883825964E-17, 1.000000000000000000 ) ) ;
#1487=AXIS2_PLACEMENT_3D ( 'NONE', #3001, #1485, #3107 ) ;
#1499=EDGE_CURVE ( 'NONE', #12966, #5103, #3092, .T. ) ;
#1508=AXIS2_PLACEMENT_3D ( 'NONE', #16904, #13343, #16588 ) ;
#1512=AXIS2_PLACEMENT_3D ( 'NONE', #3268, #9843, #16788 ) ;
#1514=ADVANCED_FACE ( 'NONE', ( #7845 ), #14474, .T. ) ;
#1518=B_SPLINE_CURVE_WITH_KNOTS ( 'NONE', 3,
 ( #310, #16641, #1826, #1601, #8396, #206, #5361, #19980, #20192, #18561, #11756, #3744, #6772, #6879, #21389, #10331 ),
 .UNSPECIFIED., .F., .F.,
 ( 4, 2, 2, 2, 2, 2, 2, 4 ),
 ( 0.02505096243559567018, 0.02646409050993621045, 0.02787721858427674726, 0.03070347473295781046, 0.03211660280729834727, 0.03352973088163888060, 0.03494285895597940700, 0.03635598703031994033 ),
 .UNSPECIFIED. ) ;
#1521=ORIENTED_EDGE ( 'NONE', *, *, #16647, .F. ) ;
#1523=EDGE_CURVE ( 'NONE', #16345, #880, #4712, .T. ) ;
#1524=VERTEX_POINT ( 'NONE', #9683 ) ;
#1525=EDGE_LOOP ( 'NONE', ( #188, #9196 ) ) ;
#1526=ORIENTED_EDGE ( 'NONE', *, *, #9290, .F. ) ;
#1537=DIRECTION ( 'NONE',  ( 0.000000000000000000, 0.000000000000000000, -1.000000000000000000 ) ) ;
#1539=CYLINDRICAL_SURFACE ( 'NONE', #18429, 125.0000000000000000 ) ;
#1541=CARTESIAN_POINT ( 'NONE',  ( -33.84809828339280102, 56.08479096960711985, 120.3299889578561590 ) ) ;
#1543=CARTESIAN_POINT ( 'NONE',  ( 107.6674317086782935, 187.4856410316723441, 20.00000000000000355 ) ) ;
#1552=ORIENTED_EDGE ( 'NONE', *, *, #11957, .T. ) ;
#1553=CARTESIAN_POINT ( 'NONE',  ( -18.68588794268873698, 323.8848358243226357, -20.00000000000000355 ) ) ;
#1562=CARTESIAN_POINT ( 'NONE',  ( 20.42502041961813930, 230.5765313837437418, -60.00000000000000000 ) ) ;
#1564=CARTESIAN_POINT ( 'NONE',  ( -26.84549718169330035, 46.23287705007100357, 49.56899837170070811 ) ) ;
#1566=PLANE ( 'NONE',  #2210 ) ;
#1569=EDGE_CURVE ( 'NONE', #8426, #17432, #4112, .T. ) ;
#1570=DIRECTION ( 'NONE',  ( -0.000000000000000000, -0.000000000000000000, 1.000000000000000000 ) ) ;
#1574=EDGE_CURVE ( 'NONE', #10312, #4551, #4700, .T. ) ;
#1580=VERTEX_POINT ( 'NONE', #6972 ) ;
#1583=EDGE_CURVE ( 'NONE', #17507, #10230, #5395, .T. ) ;
#1584=VERTEX_POINT ( 'NONE', #15427 ) ;
#1589=DIRECTION ( 'NONE',  ( -0.000000000000000000, -0.000000000000000000, 1.000000000000000000 ) ) ;
#1594=DIRECTION ( 'NONE',  ( 1.374938938973709817E-16, -1.000000000000000000, 0.000000000000000000 ) ) ;
#1595=CARTESIAN_POINT ( 'NONE',  ( 35.96497763894178945, 171.2213544847811875, -40.00000000000000000 ) ) ;
#1601=CARTESIAN_POINT ( 'NONE',  ( -30.17610990746410593, 48.40110735202731718, -49.57983718523864525 ) ) ;
#1612=ORIENTED_EDGE ( 'NONE', *, *, #10926, .F. ) ;
#1615=AXIS2_PLACEMENT_3D ( 'NONE', #7084, #16849, #18241 ) ;
#1622=EDGE_CURVE ( 'NONE', #20443, #21097, #12171, .T. ) ;
#1623=VECTOR ( 'NONE', #9251, 1000.000000000000000 ) ;
#1624=DIRECTION ( 'NONE',  ( -0.000000000000000000, 1.000000000000000000, -0.000000000000000000 ) ) ;
#1634=CARTESIAN_POINT ( 'NONE',  ( 105.7989814974898479, 142.5259582928263455, -40.00000000000000000 ) ) ;
#1635=ORIENTED_EDGE ( 'NONE', *, *, #6501, .F. ) ;
#1639=ADVANCED_FACE ( 'NONE', ( #17362 ), #4374, .F. ) ;
#1648=CARTESIAN_POINT ( 'NONE',  ( 52.60622592008805043, 30.52886280891152282, -151.0302712373927250 ) ) ;
#1675=CARTESIAN_POINT ( 'NONE',  ( -11.33448572641403906, 53.24576043933482339, 46.46721659624293466 ) ) ;
#1677=DIRECTION ( 'NONE',  ( 1.000000000000000000, 0.000000000000000000, -0.000000000000000000 ) ) ;
#1680=DIRECTION ( 'NONE',  ( 0.02283316540262222277, -0.9997392892938120612, -0.000000000000000000 ) ) ;
#1686=VECTOR ( 'NONE', #12723, 1000.000000000000000 ) ;
#1691=( BOUNDED_CURVE ( )  B_SPLINE_CURVE ( 3, ( #8667, #10181, #15291, #15395 ),
 .UNSPECIFIED., .F., .T. ) 
 B_SPLINE_CURVE_WITH_KNOTS ( ( 4, 4 ),
 ( 3.164427803482926738, 4.453488305187281782 ),
 .UNSPECIFIED. ) 
 CURVE ( )  GEOMETRIC_REPRESENTATION_ITEM ( )  RATIONAL_B_SPLINE_CURVE ( ( 1.000000000000000000, 0.8662547274802335773, 0.8662547274802335773, 1.000000000000000000 ) ) 
 REPRESENTATION_ITEM ( '' )  );
#1694=ORIENTED_EDGE ( 'NONE', *, *, #5982, .T. ) ;
#1700=CARTESIAN_POINT ( 'NONE',  ( -24.08721141673526489, 45.45117433463647671, -49.38795028004579990 ) ) ;
#1701=ADVANCED_FACE ( 'NONE', ( #1244 ), #11067, .T. ) ;
#1708=CARTESIAN_POINT ( 'NONE',  ( -28.68588794268873698, 56.85652257517428865, 0.000000000000000000 ) ) ;
#1709=CARTESIAN_POINT ( 'NONE',  ( 35.96497763894178945, 171.2213544847811875, 40.00000000000000000 ) ) ;
#1719=VECTOR ( 'NONE', #13753, 1000.000000000000000 ) ;
#1720=ORIENTED_EDGE ( 'NONE', *, *, #18947, .T. ) ;
#1724=ORIENTED_EDGE ( 'NONE', *, *, #9819, .T. ) ;
#1734=VECTOR ( 'NONE', #20383, 1000.000000000000000 ) ;
#1736=DIRECTION ( 'NONE',  ( 0.000000000000000000, 0.000000000000000000, -1.000000000000000000 ) ) ;
#1749=EDGE_CURVE ( 'NONE', #534, #16560, #6200, .T. ) ;
#1767=VECTOR ( 'NONE', #17389, 1000.000000000000000 ) ;
#1779=LINE ( 'NONE', #3064, #14329 ) ;
#1780=EDGE_CURVE ( 'NONE', #3413, #8877, #19299, .T. ) ;
#1790=CARTESIAN_POINT ( 'NONE',  ( 30.42502041961814996, 180.1716627696692967, 20.00000000000000355 ) ) ;
#1792=PLANE ( 'NONE',  #7361 ) ;
#1795=AXIS2_PLACEMENT_3D ( 'NONE', #14944, #16457, #6701 ) ;
#1801=CARTESIAN_POINT ( 'NONE',  ( -23.81231864750899874, 45.39031082328558853, -122.7132075424382975 ) ) ;
#1804=ORIENTED_EDGE ( 'NONE', *, *, #440, .F. ) ;
#1809=EDGE_CURVE ( 'NONE', #3125, #16161, #3183, .T. ) ;
#1810=CARTESIAN_POINT ( 'NONE',  ( 20.42502041961813575, 271.1055109169419666, 20.00000000000000355 ) ) ;
#1816=CARTESIAN_POINT ( 'NONE',  ( -162.2727221670389781, 30.52886280891152282, 0.000000000000000000 ) ) ;
#1820=FACE_OUTER_BOUND ( 'NONE', #12158, .T. ) ;
#1821=CARTESIAN_POINT ( 'NONE',  ( -28.68588794268873698, 10.52886280891152104, 49.60091809715359545 ) ) ;
#1826=CARTESIAN_POINT ( 'NONE',  ( -29.45535109478274549, 47.78365127927891365, -49.59625936778542155 ) ) ;
#1831=CARTESIAN_POINT ( 'NONE',  ( 65.85920792673738333, 160.1716627696692683, 20.00000000000000355 ) ) ;
#1834=CARTESIAN_POINT ( 'NONE',  ( 78.68120802659203150, 149.7457237375499517, 94.99999999999994316 ) ) ;
#1836=EDGE_CURVE ( 'NONE', #13685, #16081, #21242, .T. ) ;
#1839=CARTESIAN_POINT ( 'NONE',  ( 71.23374292195468627, 79.16544270676153872, -94.99999999999994316 ) ) ;
#1840=ADVANCED_FACE ( 'NONE', ( #19613 ), #21029, .T. ) ;
#1858=VERTEX_POINT ( 'NONE', #4586 ) ;
#1862=CIRCLE ( 'NONE', #3905, 9.999999999999994671 ) ;
#1864=ORIENTED_EDGE ( 'NONE', *, *, #2046, .F. ) ;
#1873=CARTESIAN_POINT ( 'NONE',  ( -32.29827456146021092, 51.03054495308385441, 120.7560062544352775 ) ) ;
#1874=DIRECTION ( 'NONE',  ( -0.000000000000000000, -0.000000000000000000, -1.000000000000000000 ) ) ;
#1875=DIRECTION ( 'NONE',  ( -0.1238475123623134638, 0.9177839099959486102, 0.3772724323803887114 ) ) ;
#1877=CARTESIAN_POINT ( 'NONE',  ( 60.03793209889851568, 30.52886280891152282, -131.1729372809869005 ) ) ;
#1878=AXIS2_PLACEMENT_3D ( 'NONE', #20409, #18665, #3544 ) ;
#1881=VERTEX_POINT ( 'NONE', #2974 ) ;
#1886=ORIENTED_EDGE ( 'NONE', *, *, #15142, .T. ) ;
#1899=FACE_OUTER_BOUND ( 'NONE', #16616, .T. ) ;
#1902=CIRCLE ( 'NONE', #15023, 125.0000000000000000 ) ;
#1904=LINE ( 'NONE', #3080, #947 ) ;
#1905=DIRECTION ( 'NONE',  ( 1.000000000000000000, 0.000000000000000000, 0.000000000000000000 ) ) ;
#1907=ADVANCED_FACE ( 'NONE', ( #9552 ), #17880, .F. ) ;
#1917=ORIENTED_EDGE ( 'NONE', *, *, #1923, .T. ) ;
#1918=DIRECTION ( 'NONE',  ( 0.000000000000000000, 0.000000000000000000, -1.000000000000000000 ) ) ;
#1920=VERTEX_POINT ( 'NONE', #12920 ) ;
#1922=CARTESIAN_POINT ( 'NONE',  ( -26.10681151960807611, 45.95627095229274772, -49.53444519767779752 ) ) ;
#1923=EDGE_CURVE ( 'NONE', #3984, #5712, #20048, .T. ) ;
#1925=FACE_OUTER_BOUND ( 'NONE', #4549, .T. ) ;
#1926=CARTESIAN_POINT ( 'NONE',  ( 6.416697501590670427, 172.9933428177121471, -45.00000000000000000 ) ) ;
#1928=DIRECTION ( 'NONE',  ( 0.000000000000000000, 0.000000000000000000, -1.000000000000000000 ) ) ;
#1941=ORIENTED_EDGE ( 'NONE', *, *, #14730, .T. ) ;
#1957=DIRECTION ( 'NONE',  ( 0.000000000000000000, 1.000000000000000000, 0.000000000000000000 ) ) ;
#1958=ORIENTED_EDGE ( 'NONE', *, *, #1583, .F. ) ;
#1966=ADVANCED_FACE ( 'NONE', ( #5225 ), #13352, .F. ) ;
#1971=EDGE_CURVE ( 'NONE', #8699, #13316, #1399, .T. ) ;
#1972=VECTOR ( 'NONE', #15412, 1000.000000000000114 ) ;
#1982=EDGE_CURVE ( 'NONE', #1165, #11758, #16256, .T. ) ;
#1985=ORIENTED_EDGE ( 'NONE', *, *, #3021, .F. ) ;
#1990=EDGE_LOOP ( 'NONE', ( #11807, #14723, #7245, #9725, #847, #446, #5765, #1066, #1635, #898, #9045, #9093, #16986, #2971, #7661, #12828, #15871, #17451, #18057, #7387, #6965, #3861, #3418, #2324, #9228, #8611 ) ) ;
#1991=FACE_OUTER_BOUND ( 'NONE', #18934, .T. ) ;
#1994=AXIS2_PLACEMENT_3D ( 'NONE', #16072, #16178, #18981 ) ;
#2001=DIRECTION ( 'NONE',  ( 0.000000000000000000, -1.000000000000000000, 0.000000000000000000 ) ) ;
#2003=CYLINDRICAL_SURFACE ( 'NONE', #20003, 5.000000000000004441 ) ;
#2006=DIRECTION ( 'NONE',  ( -0.000000000000000000, -0.000000000000000000, 1.000000000000000000 ) ) ;
#2011=CIRCLE ( 'NONE', #4057, 40.00000000000000000 ) ;
#2016=EDGE_LOOP ( 'NONE', ( #12187, #20247 ) ) ;
#2018=ORIENTED_EDGE ( 'NONE', *, *, #9858, .T. ) ;
#2028=CARTESIAN_POINT ( 'NONE',  ( -28.68588794268872633, 250.8848358243226357, 0.000000000000000000 ) ) ;
#2037=ORIENTED_EDGE ( 'NONE', *, *, #21318, .T. ) ;
#2042=LINE ( 'NONE', #17070, #4161 ) ;
#2046=EDGE_CURVE ( 'NONE', #12320, #10687, #11847, .T. ) ;
#2060=ORIENTED_EDGE ( 'NONE', *, *, #8116, .F. ) ;
#2063=VECTOR ( 'NONE', #19720, 1000.000000000000000 ) ;
#2065=DIRECTION ( 'NONE',  ( -0.000000000000000000, -0.000000000000000000, -1.000000000000000000 ) ) ;
#2071=DIRECTION ( 'NONE',  ( -0.000000000000000000, -0.000000000000000000, -1.000000000000000000 ) ) ;
#2086=VERTEX_POINT ( 'NONE', #5010 ) ;
#2102=LINE ( 'NONE', #18423, #9341 ) ;
#2111=CARTESIAN_POINT ( 'NONE',  ( -30.95961475400111240, 49.18261979607746071, -121.1065849196700128 ) ) ;
#2114=ORIENTED_EDGE ( 'NONE', *, *, #3555, .T. ) ;
#2126=LINE ( 'NONE', #514, #8599 ) ;
#2143=ADVANCED_FACE ( 'NONE', ( #4751 ), #7988, .F. ) ;
#2147=CARTESIAN_POINT ( 'NONE',  ( 91.21585410611801592, 56.85652257517428865, 94.99999999999994316 ) ) ;
#2158=DIRECTION ( 'NONE',  ( 0.000000000000000000, 0.000000000000000000, -1.000000000000000000 ) ) ;
#2166=ORIENTED_EDGE ( 'NONE', *, *, #1295, .F. ) ;
#2167=ORIENTED_EDGE ( 'NONE', *, *, #1499, .F. ) ;
#2181=CARTESIAN_POINT ( 'NONE',  ( -25.29117952274775760, 45.70212558035238715, 122.4152406641337478 ) ) ;
#2184=EDGE_CURVE ( 'NONE', #18163, #3421, #21368, .T. ) ;
#2203=CARTESIAN_POINT ( 'NONE',  ( 43.53705524234220547, -133.1434774248255906, 96.62835994548002816 ) ) ;
#2206=VECTOR ( 'NONE', #9331, 1000.000000000000000 ) ;
#2207=CARTESIAN_POINT ( 'NONE',  ( 20.42502041961813930, 230.5765313837437418, -60.00000000000000000 ) ) ;
#2209=CARTESIAN_POINT ( 'NONE',  ( 60.69669829156632090, 56.85652257517428865, 94.99999999999994316 ) ) ;
#2210=AXIS2_PLACEMENT_3D ( 'NONE', #16391, #16495, #1677 ) ;
#2213=CARTESIAN_POINT ( 'NONE',  ( 88.28695088269886071, 152.5259582928263740, 40.00000000000000000 ) ) ;
#2218=ORIENTED_EDGE ( 'NONE', *, *, #16102, .F. ) ;
#2222=LINE ( 'NONE', #5664, #12075 ) ;
#2227=EDGE_LOOP ( 'NONE', ( #20176, #21132, #15797, #15370 ) ) ;
#2230=AXIS2_PLACEMENT_3D ( 'NONE', #3177, #7912, #9650 ) ;
#2231=ADVANCED_FACE ( 'NONE', ( #4548 ), #17943, .T. ) ;
#2234=CARTESIAN_POINT ( 'NONE',  ( -28.68588794268872633, 250.8848358243226357, 0.000000000000000000 ) ) ;
#2254=EDGE_LOOP ( 'NONE', ( #9996, #8480, #4752, #16169 ) ) ;
#2264=CARTESIAN_POINT ( 'NONE',  ( 27.98965548446208373, 333.8848358243226357, 40.00000000000000000 ) ) ;
#2276=ORIENTED_EDGE ( 'NONE', *, *, #6973, .T. ) ;
#2280=EDGE_CURVE ( 'NONE', #17485, #9372, #9411, .T. ) ;
#2284=CARTESIAN_POINT ( 'NONE',  ( 35.96497763894179656, 163.7662197624121632, -60.00000000000000000 ) ) ;
#2289=CARTESIAN_POINT ( 'NONE',  ( 20.42502041961813575, 271.1055109169419666, 40.00000000000000000 ) ) ;
#2295=EDGE_CURVE ( 'NONE', #21097, #1920, #20562, .T. ) ;
#2296=VERTEX_POINT ( 'NONE', #19787 ) ;
#2298=VERTEX_POINT ( 'NONE', #16128 ) ;
#2302=VECTOR ( 'NONE', #11935, 1000.000000000000000 ) ;
#2308=ADVANCED_FACE ( 'NONE', ( #6265 ), #12881, .F. ) ;
#2317=LINE ( 'NONE', #7269, #243 ) ;
#2318=VECTOR ( 'NONE', #15414, 1000.000000000000000 ) ;
#2320=CARTESIAN_POINT ( 'NONE',  ( -25.27370346574498683, 45.69746946563440559, -122.4188501256071220 ) ) ;
#2324=ORIENTED_EDGE ( 'NONE', *, *, #17545, .T. ) ;
#2328=DIRECTION ( 'NONE',  ( 1.000000000000000000, 0.000000000000000000, 0.000000000000000000 ) ) ;
#2331=ORIENTED_EDGE ( 'NONE', *, *, #7194, .F. ) ;
#2336=FACE_BOUND ( 'NONE', #2016, .T. ) ;
#2337=DIRECTION ( 'NONE',  ( -0.000000000000000000, -1.000000000000000000, -0.000000000000000000 ) ) ;
#2342=DIRECTION ( 'NONE',  ( 1.000000000000000000, 0.000000000000000000, 8.901024030850960568E-17 ) ) ;
#2345=DIRECTION ( 'NONE',  ( -0.000000000000000000, -0.000000000000000000, 1.000000000000000000 ) ) ;
#2353=EDGE_CURVE ( 'NONE', #17195, #739, #12770, .T. ) ;
#2354=ADVANCED_FACE ( 'NONE', ( #14722 ), #6474, .T. ) ;
#2358=ORIENTED_EDGE ( 'NONE', *, *, #13730, .F. ) ;
#2362=CARTESIAN_POINT ( 'NONE',  ( 64.58676821086662301, 170.1716627696692683, 57.64290030256307062 ) ) ;
#2364=EDGE_CURVE ( 'NONE', #10498, #15904, #14667, .T. ) ;
#2366=FACE_OUTER_BOUND ( 'NONE', #20349, .T. ) ;
#2371=CARTESIAN_POINT ( 'NONE',  ( -22.30770786884145451, -343.0245277843623057, -122.9933582338429687 ) ) ;
#2382=ORIENTED_EDGE ( 'NONE', *, *, #13800, .F. ) ;
#2391=VECTOR ( 'NONE', #6626, 1000.000000000000000 ) ;
#2392=DIRECTION ( 'NONE',  ( 0.000000000000000000, 0.000000000000000000, -1.000000000000000000 ) ) ;
#2397=ORIENTED_EDGE ( 'NONE', *, *, #21201, .T. ) ;
#2401=ORIENTED_EDGE ( 'NONE', *, *, #4850, .T. ) ;
#2405=CARTESIAN_POINT ( 'NONE',  ( 20.42502041961813930, 230.5765313837437418, -49.99999999999999289 ) ) ;
#2408=AXIS2_PLACEMENT_3D ( 'NONE', #3130, #1404, #3240 ) ;
#2417=CARTESIAN_POINT ( 'NONE',  ( 69.55855958429435759, 152.5125485459294623, 64.92624364808513349 ) ) ;
#2419=DIRECTION ( 'NONE',  ( 0.000000000000000000, 0.000000000000000000, 1.000000000000000000 ) ) ;
#2423=DIRECTION ( 'NONE',  ( -1.000000000000000000, 0.000000000000000000, 0.000000000000000000 ) ) ;
#2432=AXIS2_PLACEMENT_3D ( 'NONE', #9762, #19404, #16171 ) ;
#2436=DIRECTION ( 'NONE',  ( 1.000000000000000000, 0.000000000000000000, 0.000000000000000000 ) ) ;
#2438=ORIENTED_EDGE ( 'NONE', *, *, #3669, .T. ) ;
#2440=CARTESIAN_POINT ( 'NONE',  ( 69.79185940953689737, 142.2976266388001250, 69.11456258820065557 ) ) ;
#2446=EDGE_CURVE ( 'NONE', #9937, #182, #19895, .T. ) ;
#2447=CIRCLE ( 'NONE', #14538, 125.0000000000000000 ) ;
#2448=LINE ( 'NONE', #5678, #9563 ) ;
#2449=CARTESIAN_POINT ( 'NONE',  ( 10.41669750159067220, 217.7548513357008630, 60.00000000000000000 ) ) ;
#2459=ORIENTED_EDGE ( 'NONE', *, *, #11869, .F. ) ;
#2462=ORIENTED_EDGE ( 'NONE', *, *, #7649, .T. ) ;
#2465=ORIENTED_EDGE ( 'NONE', *, *, #1622, .T. ) ;
#2468=CARTESIAN_POINT ( 'NONE',  ( 69.79185940953689737, 142.2976266388001250, -69.11456258820064136 ) ) ;
#2481=EDGE_CURVE ( 'NONE', #19827, #7658, #18157, .T. ) ;
#2484=ORIENTED_EDGE ( 'NONE', *, *, #14921, .T. ) ;
#2490=AXIS2_PLACEMENT_3D ( 'NONE', #11203, #6119, #7841 ) ;
#2501=DIRECTION ( 'NONE',  ( 1.374938938973709817E-16, -1.000000000000000000, 0.000000000000000000 ) ) ;
#2503=ORIENTED_EDGE ( 'NONE', *, *, #9742, .F. ) ;
#2506=VERTEX_POINT ( 'NONE', #3769 ) ;
#2509=ORIENTED_EDGE ( 'NONE', *, *, #16551, .T. ) ;
#2518=VECTOR ( 'NONE', #8598, 1000.000000000000000 ) ;
#2539=DIRECTION ( 'NONE',  ( 0.000000000000000000, 1.000000000000000000, 0.000000000000000000 ) ) ;
#2541=ORIENTED_EDGE ( 'NONE', *, *, #12879, .T. ) ;
#2546=CYLINDRICAL_SURFACE ( 'NONE', #20699, 4.000000000000001776 ) ;
#2548=CARTESIAN_POINT ( 'NONE',  ( 40.42502041961814996, 180.1716627696692967, -40.00000000000000000 ) ) ;
#2550=AXIS2_PLACEMENT_3D ( 'NONE', #3376, #13110, #20134 ) ;
#2551=EDGE_CURVE ( 'NONE', #19677, #7489, #18797, .T. ) ;
#2569=ORIENTED_EDGE ( 'NONE', *, *, #10096, .T. ) ;
#2574=FACE_OUTER_BOUND ( 'NONE', #10637, .T. ) ;
#2577=CARTESIAN_POINT ( 'NONE',  ( 20.42502041961813575, 271.1055109169419666, 40.00000000000000000 ) ) ;
#2580=LINE ( 'NONE', #754, #4557 ) ;
#2587=DIRECTION ( 'NONE',  ( 0.000000000000000000, 0.000000000000000000, 1.000000000000000000 ) ) ;
#2590=DIRECTION ( 'NONE',  ( 1.000000000000000000, 0.000000000000000000, 0.000000000000000000 ) ) ;
#2597=ORIENTED_EDGE ( 'NONE', *, *, #20952, .T. ) ;
#2606=DIRECTION ( 'NONE',  ( 0.000000000000000000, -0.000000000000000000, -1.000000000000000000 ) ) ;
#2642=FACE_BOUND ( 'NONE', #18140, .T. ) ;
#2643=VECTOR ( 'NONE', #2908, 1000.000000000000000 ) ;
#2645=LINE ( 'NONE', #12274, #5876 ) ;
#2646=DIRECTION ( 'NONE',  ( -0.000000000000000000, -0.000000000000000000, -1.000000000000000000 ) ) ;
#2648=ORIENTED_EDGE ( 'NONE', *, *, #14352, .F. ) ;
#2650=CARTESIAN_POINT ( 'NONE',  ( 51.50493485826542894, 160.1716627696692683, 61.61851857202071869 ) ) ;
#2653=CARTESIAN_POINT ( 'NONE',  ( 118.4271928232701043, -343.0245277843623057, 40.00000000000000000 ) ) ;
#2656=CIRCLE ( 'NONE', #4033, 9.999999999999994671 ) ;
#2657=DIRECTION ( 'NONE',  ( -0.000000000000000000, -0.000000000000000000, -1.000000000000000000 ) ) ;
#2660=VECTOR ( 'NONE', #2769, 1000.000000000000000 ) ;
#2666=ORIENTED_EDGE ( 'NONE', *, *, #16431, .F. ) ;
#2670=EDGE_CURVE ( 'NONE', #7489, #7633, #12316, .T. ) ;
#2671=VECTOR ( 'NONE', #12923, 1000.000000000000000 ) ;
#2672=ORIENTED_EDGE ( 'NONE', *, *, #10059, .T. ) ;
#2677=DIRECTION ( 'NONE',  ( 0.000000000000000000, 1.000000000000000000, -0.000000000000000000 ) ) ;
#2681=ADVANCED_FACE ( 'NONE', ( #12424 ), #17086, .T. ) ;
#2686=CARTESIAN_POINT ( 'NONE',  ( 30.42502041961813575, 271.1055109169419097, -20.00000000000000355 ) ) ;
#2692=EDGE_CURVE ( 'NONE', #12017, #6673, #15467, .T. ) ;
#2696=AXIS2_PLACEMENT_3D ( 'NONE', #6582, #19360, #4651 ) ;
#2701=ORIENTED_EDGE ( 'NONE', *, *, #7215, .F. ) ;
#2702=VERTEX_POINT ( 'NONE', #8943 ) ;
#2715=ADVANCED_FACE ( 'NONE', ( #14269 ), #20958, .F. ) ;
#2718=DIRECTION ( 'NONE',  ( 0.000000000000000000, -1.000000000000000000, 0.000000000000000000 ) ) ;
#2724=ORIENTED_EDGE ( 'NONE', *, *, #7962, .T. ) ;
#2726=ORIENTED_EDGE ( 'NONE', *, *, #2353, .F. ) ;
#2727=LINE ( 'NONE', #21210, #17359 ) ;
#2735=AXIS2_PLACEMENT_3D ( 'NONE', #16601, #11388, #7923 ) ;
#2737=CARTESIAN_POINT ( 'NONE',  ( -28.68588794268872633, 174.3162933293988033, 0.000000000000000000 ) ) ;
#2742=DIRECTION ( 'NONE',  ( 0.000000000000000000, -0.9253149302858357794, -0.3791995250394160633 ) ) ;
#2753=DIRECTION ( 'NONE',  ( 1.000000000000000000, 0.000000000000000000, 0.000000000000000000 ) ) ;
#2769=DIRECTION ( 'NONE',  ( -1.374938938973709817E-16, 1.000000000000000000, 0.000000000000000000 ) ) ;
#2770=CARTESIAN_POINT ( 'NONE',  ( 125.7989814974898053, 10.52886280891152104, 40.00000000000000000 ) ) ;
#2775=CARTESIAN_POINT ( 'NONE',  ( 105.7989814974898479, 142.5259582928263455, -20.00000000000000355 ) ) ;
#2785=VERTEX_POINT ( 'NONE', #7532 ) ;
#2789=FACE_OUTER_BOUND ( 'NONE', #11656, .T. ) ;
#2792=FACE_BOUND ( 'NONE', #3520, .T. ) ;
#2794=PLANE ( 'NONE',  #5248 ) ;
#2802=EDGE_CURVE ( 'NONE', #12320, #1316, #19007, .T. ) ;
#2806=DIRECTION ( 'NONE',  ( 1.000000000000000000, 0.000000000000000000, 0.000000000000000000 ) ) ;
#2807=ORIENTED_EDGE ( 'NONE', *, *, #13252, .T. ) ;
#2833=AXIS2_PLACEMENT_3D ( 'NONE', #6354, #1396, #4837 ) ;
#2835=CARTESIAN_POINT ( 'NONE',  ( 91.21585410611801592, 31.85652257517428865, -85.46735025547123143 ) ) ;
#2850=PLANE ( 'NONE',  #15774 ) ;
#2856=ORIENTED_EDGE ( 'NONE', *, *, #17543, .F. ) ;
#2858=VERTEX_POINT ( 'NONE', #1595 ) ;
#2859=VECTOR ( 'NONE', #18979, 1000.000000000000114 ) ;
#2870=DIRECTION ( 'NONE',  ( -0.000000000000000000, 1.000000000000000000, -0.000000000000000000 ) ) ;
#2873=PLANE ( 'NONE',  #20135 ) ;
#2877=ADVANCED_FACE ( 'NONE', ( #4515 ), #14584, .F. ) ;
#2882=VERTEX_POINT ( 'NONE', #4936 ) ;
#2889=VECTOR ( 'NONE', #5929, 1000.000000000000000 ) ;
#2895=ORIENTED_EDGE ( 'NONE', *, *, #9613, .T. ) ;
#2896=CARTESIAN_POINT ( 'NONE',  ( 6.416697501590670427, 172.9933428177121471, 60.00000000000000000 ) ) ;
#2897=CARTESIAN_POINT ( 'NONE',  ( 2.416697501590669095, 172.9933428177121471, 45.00000000000000000 ) ) ;
#2898=EDGE_CURVE ( 'NONE', #15497, #15607, #6658, .T. ) ;
#2900=DIRECTION ( 'NONE',  ( -1.000000000000000000, 0.000000000000000000, 0.000000000000000000 ) ) ;
#2906=ADVANCED_FACE ( 'NONE', ( #14799 ), #6549, .F. ) ;
#2907=VECTOR ( 'NONE', #19983, 1000.000000000000000 ) ;
#2908=DIRECTION ( 'NONE',  ( -0.000000000000000000, -0.000000000000000000, 1.000000000000000000 ) ) ;
#2915=CARTESIAN_POINT ( 'NONE',  ( 60.03793209889851568, 10.52886280891152104, -136.1729372809869005 ) ) ;
#2928=LINE ( 'NONE', #7674, #14204 ) ;
#2931=CARTESIAN_POINT ( 'NONE',  ( 29.72350413846044859, 280.4463447002762564, -40.00000000000000000 ) ) ;
#2932=ORIENTED_EDGE ( 'NONE', *, *, #1483, .F. ) ;
#2935=ORIENTED_EDGE ( 'NONE', *, *, #7105, .F. ) ;
#2936=VERTEX_POINT ( 'NONE', #6441 ) ;
#2940=EDGE_CURVE ( 'NONE', #9142, #15603, #7954, .T. ) ;
#2942=DIRECTION ( 'NONE',  ( 1.000000000000000000, 0.000000000000000000, 0.000000000000000000 ) ) ;
#2953=DIRECTION ( 'NONE',  ( 1.250996701150283068E-16, -1.000000000000000000, 0.000000000000000000 ) ) ;
#2954=DIRECTION ( 'NONE',  ( 1.000000000000000000, 0.000000000000000000, 0.000000000000000000 ) ) ;
#2955=DIRECTION ( 'NONE',  ( 1.000000000000000000, 0.000000000000000000, -0.000000000000000000 ) ) ;
#2963=VERTEX_POINT ( 'NONE', #8063 ) ;
#2966=EDGE_CURVE ( 'NONE', #15904, #182, #17911, .T. ) ;
#2971=ORIENTED_EDGE ( 'NONE', *, *, #14654, .T. ) ;
#2974=CARTESIAN_POINT ( 'NONE',  ( 71.23374292195467206, 79.16544270676152451, 94.99999999999994316 ) ) ;
#2976=CARTESIAN_POINT ( 'NONE',  ( -25.61611216564576665, 45.79743936472188182, 49.50645936902517263 ) ) ;
#2984=LINE ( 'NONE', #4699, #1623 ) ;
#2986=ORIENTED_EDGE ( 'NONE', *, *, #11157, .F. ) ;
#2997=VECTOR ( 'NONE', #21329, 1000.000000000000000 ) ;
#3001=CARTESIAN_POINT ( 'NONE',  ( -49.57497958038186425, 230.5765313837437418, 49.99999999999999289 ) ) ;
#3002=CARTESIAN_POINT ( 'NONE',  ( -22.30770786884145451, 30.52886280891152282, 122.9933582338429972 ) ) ;
#3014=VECTOR ( 'NONE', #8793, 1000.000000000000000 ) ;
#3015=PLANE ( 'NONE',  #6328 ) ;
#3021=EDGE_CURVE ( 'NONE', #258, #10312, #4626, .T. ) ;
#3032=PRODUCT_DEFINITION_SHAPE ( 'NONE', 'NONE',  #15858 ) ;
#3038=ORIENTED_EDGE ( 'NONE', *, *, #21080, .F. ) ;
#3043=FACE_OUTER_BOUND ( 'NONE', #5845, .T. ) ;
#3062=DIRECTION ( 'NONE',  ( 0.000000000000000000, -1.000000000000000000, 0.000000000000000000 ) ) ;
#3064=CARTESIAN_POINT ( 'NONE',  ( 40.42502041961814996, 170.1716627696692683, -20.00000000000000355 ) ) ;
#3078=DIRECTION ( 'NONE',  ( 0.000000000000000000, 0.000000000000000000, -1.000000000000000000 ) ) ;
#3080=CARTESIAN_POINT ( 'NONE',  ( 71.32175588950862277, 75.31183677523708297, -94.99999999999994316 ) ) ;
#3089=EDGE_LOOP ( 'NONE', ( #16242, #14565, #17246, #12295 ) ) ;
#3090=DIRECTION ( 'NONE',  ( 0.000000000000000000, 0.000000000000000000, 1.000000000000000000 ) ) ;
#3092=CIRCLE ( 'NONE', #14161, 125.0000000000000000 ) ;
#3095=EDGE_LOOP ( 'NONE', ( #18663, #20973, #2382, #1209 ) ) ;
#3100=DIRECTION ( 'NONE',  ( -0.000000000000000000, -0.000000000000000000, 1.000000000000000000 ) ) ;
#3101=VECTOR ( 'NONE', #20232, 999.9999999999998863 ) ;
#3107=DIRECTION ( 'NONE',  ( 0.000000000000000000, -1.000000000000000000, 9.855701800883825964E-17 ) ) ;
#3108=DIRECTION ( 'NONE',  ( 0.000000000000000000, -1.000000000000000000, 0.000000000000000000 ) ) ;
#3109=VECTOR ( 'NONE', #6523, 1000.000000000000000 ) ;
#3110=DIRECTION ( 'NONE',  ( 0.000000000000000000, -0.000000000000000000, 1.000000000000000000 ) ) ;
#3113=EDGE_CURVE ( 'NONE', #11304, #17379, #18237, .T. ) ;
#3114=CARTESIAN_POINT ( 'NONE',  ( 43.53705524234220547, -133.1434774248255906, -96.62835994548002816 ) ) ;
#3116=FACE_OUTER_BOUND ( 'NONE', #21153, .T. ) ;
#3125=VERTEX_POINT ( 'NONE', #1821 ) ;
#3130=CARTESIAN_POINT ( 'NONE',  ( 105.7989814974898479, 152.5259582928263740, 20.00000000000000355 ) ) ;
#3137=DIRECTION ( 'NONE',  ( -1.157565925312684532E-16, 0.9253149302858357794, -0.3791995250394160633 ) ) ;
#3138=EDGE_CURVE ( 'NONE', #9575, #16161, #4914, .T. ) ;
#3140=CARTESIAN_POINT ( 'NONE',  ( 79.78925230247502043, 142.5259582928263455, -20.00000000000000355 ) ) ;
#3141=ORIENTED_EDGE ( 'NONE', *, *, #6501, .T. ) ;
#3153=AXIS2_PLACEMENT_3D ( 'NONE', #12038, #14005, #8684 ) ;
#3158=ADVANCED_FACE ( 'NONE', ( #21127 ), #8125, .F. ) ;
#3162=CARTESIAN_POINT ( 'NONE',  ( 0.000000000000000000, -343.0245277843623057, 0.000000000000000000 ) ) ;
#3171=ORIENTED_EDGE ( 'NONE', *, *, #20988, .T. ) ;
#3176=EDGE_LOOP ( 'NONE', ( #13530, #14546, #13118, #14686 ) ) ;
#3177=CARTESIAN_POINT ( 'NONE',  ( 60.03793209889851568, 30.52886280891152282, -131.1729372809869005 ) ) ;
#3183=LINE ( 'NONE', #14661, #16919 ) ;
#3187=LINE ( 'NONE', #19617, #16718 ) ;
#3193=ADVANCED_FACE ( 'NONE', ( #11272 ), #9857, .T. ) ;
#3200=ORIENTED_EDGE ( 'NONE', *, *, #20326, .T. ) ;
#3204=EDGE_LOOP ( 'NONE', ( #5315, #16301, #13071, #14291, #3360 ) ) ;
#3205=DIRECTION ( 'NONE',  ( -0.000000000000000000, -0.000000000000000000, -1.000000000000000000 ) ) ;
#3209=CARTESIAN_POINT ( 'NONE',  ( 35.96497763894178945, 170.1716627696692683, 20.00000000000000355 ) ) ;
#3210=EDGE_CURVE ( 'NONE', #12803, #16558, #16162, .T. ) ;
#3213=LINE ( 'NONE', #14796, #5776 ) ;
#3217=VECTOR ( 'NONE', #4795, 1000.000000000000000 ) ;
#3225=EDGE_CURVE ( 'NONE', #14751, #13685, #1339, .T. ) ;
#3231=ORIENTED_EDGE ( 'NONE', *, *, #17240, .F. ) ;
#3235=EDGE_CURVE ( 'NONE', #6356, #19050, #1779, .T. ) ;
#3238=VECTOR ( 'NONE', #10633, 1000.000000000000000 ) ;
#3240=DIRECTION ( 'NONE',  ( -1.000000000000000000, 0.000000000000000000, 0.000000000000000000 ) ) ;
#3242=CIRCLE ( 'NONE', #14646, 10.00000000000000178 ) ;
#3248=DIRECTION ( 'NONE',  ( 1.000000000000000000, 0.000000000000000000, 0.000000000000000000 ) ) ;
#3252=DIRECTION ( 'NONE',  ( 0.000000000000000000, 0.000000000000000000, -1.000000000000000000 ) ) ;
#3254=ORIENTED_EDGE ( 'NONE', *, *, #6927, .T. ) ;
#3258=AXIS2_PLACEMENT_3D ( 'NONE', #17874, #19606, #19932 ) ;
#3268=CARTESIAN_POINT ( 'NONE',  ( -18.68588794268873698, 281.1055109169419666, -20.00000000000000355 ) ) ;
#3270=CARTESIAN_POINT ( 'NONE',  ( -33.84809828339280102, 56.85652257517428865, 120.3299889578561448 ) ) ;
#3271=DIRECTION ( 'NONE',  ( -1.000000000000000000, -0.000000000000000000, -0.000000000000000000 ) ) ;
#3272=FACE_OUTER_BOUND ( 'NONE', #9149, .T. ) ;
#3274=EDGE_CURVE ( 'NONE', #3284, #15800, #1902, .T. ) ;
#3283=CARTESIAN_POINT ( 'NONE',  ( 60.03793209889851568, 10.52886280891152104, 126.1729372809868863 ) ) ;
#3284=VERTEX_POINT ( 'NONE', #4895 ) ;
#3287=CARTESIAN_POINT ( 'NONE',  ( 60.03793209889851568, 30.52886280891152282, -152.3753892284480003 ) ) ;
#3296=CARTESIAN_POINT ( 'NONE',  ( 78.68120802659203150, 149.7457237375499517, 94.99999999999994316 ) ) ;
#3298=DIRECTION ( 'NONE',  ( 0.000000000000000000, 0.000000000000000000, -1.000000000000000000 ) ) ;
#3312=LINE ( 'NONE', #11093, #13160 ) ;
#3316=DIRECTION ( 'NONE',  ( 0.000000000000000000, -1.000000000000000000, 0.000000000000000000 ) ) ;
#3320=CARTESIAN_POINT ( 'NONE',  ( 81.24038404635965094, 10.52886280891152104, 131.1729372809869005 ) ) ;
#3325=DIRECTION ( 'NONE',  ( 1.000000000000000000, 0.000000000000000000, 0.000000000000000000 ) ) ;
#3336=EDGE_CURVE ( 'NONE', #264, #17635, #13237, .T. ) ;
#3339=LINE ( 'NONE', #17436, #17978 ) ;
#3353=EDGE_CURVE ( 'NONE', #2858, #6356, #19494, .T. ) ;
#3357=ORIENTED_EDGE ( 'NONE', *, *, #13122, .F. ) ;
#3360=ORIENTED_EDGE ( 'NONE', *, *, #10816, .F. ) ;
#3362=FACE_BOUND ( 'NONE', #16513, .T. ) ;
#3366=VECTOR ( 'NONE', #14553, 1000.000000000000000 ) ;
#3376=CARTESIAN_POINT ( 'NONE',  ( 292.4526463419396691, 308.2087638784415162, -20.00000000000000355 ) ) ;
#3385=ORIENTED_EDGE ( 'NONE', *, *, #14271, .T. ) ;
#3388=ORIENTED_EDGE ( 'NONE', *, *, #13411, .T. ) ;
#3391=DIRECTION ( 'NONE',  ( 0.000000000000000000, 0.000000000000000000, -1.000000000000000000 ) ) ;
#3399=CARTESIAN_POINT ( 'NONE',  ( -27.78321401995996709, 46.69440907075437508, 49.59323028521529153 ) ) ;
#3400=CARTESIAN_POINT ( 'NONE',  ( -49.57497958038186425, 230.5765313837437418, -49.99999999999999289 ) ) ;
#3405=CARTESIAN_POINT ( 'NONE',  ( 81.24038404635965094, 30.52886280891152282, -131.1729372809869005 ) ) ;
#3411=VECTOR ( 'NONE', #7075, 1000.000000000000000 ) ;
#3413=VERTEX_POINT ( 'NONE', #684 ) ;
#3418=ORIENTED_EDGE ( 'NONE', *, *, #17690, .T. ) ;
#3421=VERTEX_POINT ( 'NONE', #8777 ) ;
#3423=CARTESIAN_POINT ( 'NONE',  ( -16.60355223547259484, 46.82116177588022765, -48.10739902922093592 ) ) ;
#3429=CARTESIAN_POINT ( 'NONE',  ( -33.84809828339280102, 56.85652257517428865, 49.33155846391706945 ) ) ;
#3430=VECTOR ( 'NONE', #912, 1000.000000000000114 ) ;
#3431=CARTESIAN_POINT ( 'NONE',  ( 30.42502041961813575, 271.1055109169419097, 20.00000000000000355 ) ) ;
#3440=ORIENTED_EDGE ( 'NONE', *, *, #8077, .T. ) ;
#3454=EDGE_CURVE ( 'NONE', #1161, #2785, #1691, .T. ) ;
#3456=DIRECTION ( 'NONE',  ( -0.3505116388060184329, 0.000000000000000000, 0.9365583756827543516 ) ) ;
#3457=ORIENTED_EDGE ( 'NONE', *, *, #19817, .T. ) ;
#3464=DIRECTION ( 'NONE',  ( 9.855701800883827197E-17, -1.000000000000000000, 0.000000000000000000 ) ) ;
#3466=ORIENTED_EDGE ( 'NONE', *, *, #20411, .F. ) ;
#3470=ADVANCED_FACE ( 'NONE', ( #13447 ), #3598, .F. ) ;
#3471=VECTOR ( 'NONE', #2646, 1000.000000000000000 ) ;
#3473=LINE ( 'NONE', #18600, #1719 ) ;
#3475=DIRECTION ( 'NONE',  ( 0.000000000000000000, 1.000000000000000000, 0.000000000000000000 ) ) ;
#3502=DIRECTION ( 'NONE',  ( 0.000000000000000000, 1.000000000000000000, 0.000000000000000000 ) ) ;
#3505=CARTESIAN_POINT ( 'NONE',  ( 88.28695088269886071, 142.5259582928263455, -20.00000000000000355 ) ) ;
#3511=FACE_OUTER_BOUND ( 'NONE', #8929, .T. ) ;
#3517=ORIENTED_EDGE ( 'NONE', *, *, #18529, .F. ) ;
#3520=EDGE_LOOP ( 'NONE', ( #13660, #20073 ) ) ;
#3521=CIRCLE ( 'NONE', #13193, 4.000000000000001776 ) ;
#3528=CARTESIAN_POINT ( 'NONE',  ( 107.6674317086782935, 187.4856410316723441, 20.00000000000000355 ) ) ;
#3529=FACE_OUTER_BOUND ( 'NONE', #3176, .T. ) ;
#3532=ADVANCED_FACE ( 'NONE', ( #1991 ), #18720, .F. ) ;
#3534=DIRECTION ( 'NONE',  ( 1.000000000000000000, 0.000000000000000000, 0.000000000000000000 ) ) ;
#3539=DIRECTION ( 'NONE',  ( 1.000000000000000000, 0.000000000000000000, 0.000000000000000000 ) ) ;
#3543=ORIENTED_EDGE ( 'NONE', *, *, #15578, .T. ) ;
#3544=DIRECTION ( 'NONE',  ( 0.000000000000000000, -1.000000000000000000, 0.000000000000000000 ) ) ;
#3555=EDGE_CURVE ( 'NONE', #18299, #2963, #18614, .T. ) ;
#3569=ORIENTED_EDGE ( 'NONE', *, *, #8372, .T. ) ;
#3573=AXIS2_PLACEMENT_3D ( 'NONE', #764, #15580, #2590 ) ;
#3575=VERTEX_POINT ( 'NONE', #4445 ) ;
#3579=CARTESIAN_POINT ( 'NONE',  ( -10.76731745429009912, 56.85652257517428865, -118.3724535612433328 ) ) ;
#3583=CARTESIAN_POINT ( 'NONE',  ( -29.89856342657186872, 48.13176998328706446, 121.3728849402414198 ) ) ;
#3585=CARTESIAN_POINT ( 'NONE',  ( -18.68588794268873698, 281.1055109169419666, -40.00000000000000000 ) ) ;
#3590=ORIENTED_EDGE ( 'NONE', *, *, #16291, .T. ) ;
#3593=VECTOR ( 'NONE', #4192, 1000.000000000000000 ) ;
#3597=EDGE_LOOP ( 'NONE', ( #18467, #9370 ) ) ;
#3598=PLANE ( 'NONE',  #6702 ) ;
#3607=FACE_OUTER_BOUND ( 'NONE', #17222, .T. ) ;
#3617=DIRECTION ( 'NONE',  ( -3.836511174089486173E-16, 0.000000000000000000, 1.000000000000000000 ) ) ;
#3621=ORIENTED_EDGE ( 'NONE', *, *, #7962, .F. ) ;
#3624=ORIENTED_EDGE ( 'NONE', *, *, #5125, .T. ) ;
#3632=CARTESIAN_POINT ( 'NONE',  ( -27.79598376143726668, 46.69101496124648065, -49.59521087409807905 ) ) ;
#3634=CYLINDRICAL_SURFACE ( 'NONE', #18254, 22.72497359561857877 ) ;
#3637=CARTESIAN_POINT ( 'NONE',  ( 6.416697501590670427, 172.9933428177121471, -45.00000000000000000 ) ) ;
#3638=EDGE_CURVE ( 'NONE', #9753, #5025, #10707, .T. ) ;
#3651=ORIENTED_EDGE ( 'NONE', *, *, #13101, .T. ) ;
#3653=DIRECTION ( 'NONE',  ( 1.000000000000000000, 0.000000000000000000, 0.000000000000000000 ) ) ;
#3660=DIRECTION ( 'NONE',  ( -0.000000000000000000, -0.000000000000000000, 1.000000000000000000 ) ) ;
#3669=EDGE_CURVE ( 'NONE', #9372, #16429, #796, .T. ) ;
#3670=AXIS2_PLACEMENT_3D ( 'NONE', #15786, #15679, #13834 ) ;
#3674=ORIENTED_EDGE ( 'NONE', *, *, #18002, .F. ) ;
#3682=AXIS2_PLACEMENT_3D ( 'NONE', #10869, #12826, #17475 ) ;
#3687=VECTOR ( 'NONE', #20830, 1000.000000000000000 ) ;
#3698=ORIENTED_EDGE ( 'NONE', *, *, #1809, .T. ) ;
#3708=FACE_OUTER_BOUND ( 'NONE', #18774, .T. ) ;
#3712=VECTOR ( 'NONE', #411, 1000.000000000000000 ) ;
#3713=CARTESIAN_POINT ( 'NONE',  ( 20.42502041961806825, 281.1055109169419666, -20.00000000000000355 ) ) ;
#3719=CARTESIAN_POINT ( 'NONE',  ( 6.416697501590670427, 172.9933428177121471, -50.00000000000000000 ) ) ;
#3720=EDGE_CURVE ( 'NONE', #3882, #15977, #19085, .T. ) ;
#3727=EDGE_LOOP ( 'NONE', ( #1724, #19469, #12666, #12427 ) ) ;
#3730=VERTEX_POINT ( 'NONE', #17433 ) ;
#3736=DIRECTION ( 'NONE',  ( 1.000000000000000000, 0.000000000000000000, 0.000000000000000000 ) ) ;
#3739=DIRECTION ( 'NONE',  ( 0.000000000000000000, 1.000000000000000000, 0.000000000000000000 ) ) ;
#3741=CIRCLE ( 'NONE', #12392, 49.60091809715359545 ) ;
#3744=CARTESIAN_POINT ( 'NONE',  ( -33.61217542136964909, 54.48747864393421736, -49.35581280498866619 ) ) ;
#3752=LINE ( 'NONE', #16860, #5533 ) ;
#3754=EDGE_LOOP ( 'NONE', ( #11626, #9540 ) ) ;
#3761=DIRECTION ( 'NONE',  ( -0.000000000000000000, -0.000000000000000000, -1.000000000000000000 ) ) ;
#3767=CIRCLE ( 'NONE', #15881, 9.999999999999994671 ) ;
#3769=CARTESIAN_POINT ( 'NONE',  ( 30.42502041961814996, 180.1716627696692967, 40.00000000000000000 ) ) ;
#3771=ORIENTED_EDGE ( 'NONE', *, *, #15494, .F. ) ;
#3774=ORIENTED_EDGE ( 'NONE', *, *, #4850, .F. ) ;
#3777=DIRECTION ( 'NONE',  ( 1.000000000000000000, 0.000000000000000000, 0.000000000000000000 ) ) ;
#3781=AXIS2_PLACEMENT_3D ( 'NONE', #17934, #16438, #9815 ) ;
#3785=CARTESIAN_POINT ( 'NONE',  ( 88.28695088269886071, 142.5259582928263455, 40.00000000000000000 ) ) ;
#3799=EDGE_LOOP ( 'NONE', ( #15691, #8931, #10108, #9514 ) ) ;
#3800=CARTESIAN_POINT ( 'NONE',  ( 20.42502041961814641, 160.1716627696692683, 40.00000000000000000 ) ) ;
#3816=EDGE_CURVE ( 'NONE', #6145, #10102, #18042, .T. ) ;
#3823=CARTESIAN_POINT ( 'NONE',  ( -33.84809828339280102, 56.85652257517428865, -120.3299889578561448 ) ) ;
#3824=AXIS2_PLACEMENT_3D ( 'NONE', #1218, #20896, #2942 ) ;
#3827=EDGE_LOOP ( 'NONE', ( #6779, #19799, #12620, #19741 ) ) ;
#3829=EDGE_LOOP ( 'NONE', ( #14865, #11737, #16377, #12568 ) ) ;
#3831=LINE ( 'NONE', #13687, #17400 ) ;
#3838=CARTESIAN_POINT ( 'NONE',  ( -23.30663226349542327, 45.35645063453653592, -49.30906092905553351 ) ) ;
#3842=EDGE_CURVE ( 'NONE', #18961, #3882, #2727, .T. ) ;
#3848=FACE_OUTER_BOUND ( 'NONE', #14624, .T. ) ;
#3854=ORIENTED_EDGE ( 'NONE', *, *, #8963, .T. ) ;
#3861=ORIENTED_EDGE ( 'NONE', *, *, #13021, .T. ) ;
#3873=EDGE_CURVE ( 'NONE', #1165, #13817, #11141, .T. ) ;
#3881=ORIENTED_EDGE ( 'NONE', *, *, #18949, .F. ) ;
#3882=VERTEX_POINT ( 'NONE', #17746 ) ;
#3886=ORIENTED_EDGE ( 'NONE', *, *, #20255, .F. ) ;
#3895=AXIS2_PLACEMENT_3D ( 'NONE', #7348, #2718, #19045 ) ;
#3905=AXIS2_PLACEMENT_3D ( 'NONE', #12646, #10898, #17614 ) ;
#3906=EDGE_LOOP ( 'NONE', ( #14225, #475 ) ) ;
#3907=ORIENTED_EDGE ( 'NONE', *, *, #7023, .T. ) ;
#3925=DIRECTION ( 'NONE',  ( 0.000000000000000000, 0.000000000000000000, -1.000000000000000000 ) ) ;
#3926=CARTESIAN_POINT ( 'NONE',  ( 292.4526463419396691, 308.2087638784415162, 40.00000000000000000 ) ) ;
#3931=CARTESIAN_POINT ( 'NONE',  ( -32.07601836630501424, 50.69989608122271818, -120.8146399612313502 ) ) ;
#3938=CARTESIAN_POINT ( 'NONE',  ( 40.42502041961814996, 180.1716627696692967, 40.00000000000000000 ) ) ;
#3939=ADVANCED_FACE ( 'NONE', ( #3362, #13097, #11353 ), #17950, .T. ) ;
#3940=CYLINDRICAL_SURFACE ( 'NONE', #17284, 220.7252770684332006 ) ;
#3943=ORIENTED_EDGE ( 'NONE', *, *, #13996, .T. ) ;
#3949=CARTESIAN_POINT ( 'NONE',  ( 20.42502041961814641, 160.1716627696692683, -61.32762281133329907 ) ) ;
#3966=ORIENTED_EDGE ( 'NONE', *, *, #20990, .F. ) ;
#3973=LINE ( 'NONE', #20534, #20821 ) ;
#3984=VERTEX_POINT ( 'NONE', #14928 ) ;
#3997=ADVANCED_FACE ( 'NONE', ( #20107 ), #5276, .F. ) ;
#4023=CIRCLE ( 'NONE', #1615, 9.999999999999994671 ) ;
#4025=DIRECTION ( 'NONE',  ( -0.000000000000000000, 1.000000000000000000, -0.000000000000000000 ) ) ;
#4032=CARTESIAN_POINT ( 'NONE',  ( 30.42502041961813575, 271.1055109169419097, 40.00000000000000000 ) ) ;
#4033=AXIS2_PLACEMENT_3D ( 'NONE', #5160, #13499, #3539 ) ;
#4039=ORIENTED_EDGE ( 'NONE', *, *, #8948, .T. ) ;
#4044=LINE ( 'NONE', #1033, #2206 ) ;
#4046=LINE ( 'NONE', #12493, #3471 ) ;
#4048=EDGE_LOOP ( 'NONE', ( #6699, #11120, #20618, #13525 ) ) ;
#4056=CARTESIAN_POINT ( 'NONE',  ( 43.53705524234220547, 56.85652257517428865, 96.62835994548002816 ) ) ;
#4057=AXIS2_PLACEMENT_3D ( 'NONE', #7901, #12901, #17860 ) ;
#4060=PLANE ( 'NONE',  #15942 ) ;
#4063=EDGE_CURVE ( 'NONE', #4339, #6752, #1075, .T. ) ;
#4075=ORIENTED_EDGE ( 'NONE', *, *, #17946, .T. ) ;
#4083=DIRECTION ( 'NONE',  ( 1.000000000000000000, -0.000000000000000000, -0.000000000000000000 ) ) ;
#4093=ORIENTED_EDGE ( 'NONE', *, *, #1422, .T. ) ;
#4094=ORIENTED_EDGE ( 'NONE', *, *, #16856, .T. ) ;
#4099=VERTEX_POINT ( 'NONE', #5809 ) ;
#4107=CIRCLE ( 'NONE', #16215, 4.999999999999990230 ) ;
#4108=LINE ( 'NONE', #997, #16502 ) ;
#4112=CIRCLE ( 'NONE', #17930, 20.57735571454641033 ) ;
#4117=EDGE_LOOP ( 'NONE', ( #20440, #7732, #16535, #16217, #12982, #14390, #5983, #6989, #3907, #9336, #3543, #2276, #8119, #9726, #17201 ) ) ;
#4122=AXIS2_PLACEMENT_3D ( 'NONE', #7025, #11901, #11795 ) ;
#4123=EDGE_CURVE ( 'NONE', #13817, #7658, #10458, .T. ) ;
#4135=DIRECTION ( 'NONE',  ( 0.9999562017632421806, 0.000000000000000000, -0.009359196291876339252 ) ) ;
#4136=CARTESIAN_POINT ( 'NONE',  ( 52.60622592008805043, 30.52886280891152282, 151.0302712373927250 ) ) ;
#4139=DIRECTION ( 'NONE',  ( 1.232945044042657126E-32, -9.855701800883825964E-17, 1.000000000000000000 ) ) ;
#4147=DIRECTION ( 'NONE',  ( 0.000000000000000000, -0.000000000000000000, 1.000000000000000000 ) ) ;
#4148=EDGE_CURVE ( 'NONE', #20120, #6145, #3973, .T. ) ;
#4150=CARTESIAN_POINT ( 'NONE',  ( 20.42502041961813575, 271.1055109169419666, -40.00000000000000000 ) ) ;
#4161=VECTOR ( 'NONE', #8613, 1000.000000000000000 ) ;
#4171=VECTOR ( 'NONE', #15562, 1000.000000000000000 ) ;
#4174=ORIENTED_EDGE ( 'NONE', *, *, #3353, .T. ) ;
#4180=VECTOR ( 'NONE', #17889, 1000.000000000000000 ) ;
#4189=CARTESIAN_POINT ( 'NONE',  ( 20.42502041961813930, 230.5765313837437418, 49.99999999999999289 ) ) ;
#4191=CARTESIAN_POINT ( 'NONE',  ( 78.68120802659203150, 149.7457237375499517, 66.14548919766383506 ) ) ;
#4192=DIRECTION ( 'NONE',  ( -0.000000000000000000, 1.000000000000000000, -0.000000000000000000 ) ) ;
#4194=DIRECTION ( 'NONE',  ( 0.000000000000000000, 0.000000000000000000, 1.000000000000000000 ) ) ;
#4201=EDGE_CURVE ( 'NONE', #11949, #6011, #20636, .T. ) ;
#4202=ADVANCED_FACE ( 'NONE', ( #2366 ), #17496, .F. ) ;
#4204=UNCERTAINTY_MEASURE_WITH_UNIT (LENGTH_MEASURE( 1.000000000000000082E-05 ), #10723, 'distance_accuracy_value', 'NONE');
#4210=ORIENTED_EDGE ( 'NONE', *, *, #1780, .F. ) ;
#4211=VERTEX_POINT ( 'NONE', #2686 ) ;
#4215=EDGE_CURVE ( 'NONE', #880, #4398, #2580, .T. ) ;
#4227=CARTESIAN_POINT ( 'NONE',  ( 78.68120802659203150, 149.7457237375499517, -94.99999999999994316 ) ) ;
#4228=DIRECTION ( 'NONE',  ( 0.000000000000000000, -1.000000000000000000, 0.000000000000000000 ) ) ;
#4229=CARTESIAN_POINT ( 'NONE',  ( 2.416697501590669095, 172.9933428177121471, -50.00000000000000000 ) ) ;
#4231=VERTEX_POINT ( 'NONE', #13059 ) ;
#4232=AXIS2_PLACEMENT_3D ( 'NONE', #11881, #3660, #16868 ) ;
#4235=EDGE_LOOP ( 'NONE', ( #3141, #2166, #18379, #1030 ) ) ;
#4236=ORIENTED_EDGE ( 'NONE', *, *, #179, .T. ) ;
#4237=CARTESIAN_POINT ( 'NONE',  ( 81.24038404635966515, -343.0245277843623057, 94.99999999999994316 ) ) ;
#4241=FACE_OUTER_BOUND ( 'NONE', #3204, .T. ) ;
#4242=CARTESIAN_POINT ( 'NONE',  ( 91.21585410611801592, 56.85652257517428865, -40.00000000000000000 ) ) ;
#4275=DIRECTION ( 'NONE',  ( 1.000000000000000000, 0.000000000000000000, -0.000000000000000000 ) ) ;
#4276=CARTESIAN_POINT ( 'NONE',  ( 82.89408817951444064, 286.0648460576640559, 40.00000000000000000 ) ) ;
#4280=CARTESIAN_POINT ( 'NONE',  ( 28.16023193154655502, 323.8848358243226357, 20.00000000000000355 ) ) ;
#4283=ADVANCED_FACE ( 'NONE', ( #12636 ), #2794, .T. ) ;
#4296=ORIENTED_EDGE ( 'NONE', *, *, #300, .T. ) ;
#4298=DIRECTION ( 'NONE',  ( -1.000000000000000000, 0.000000000000000000, 0.000000000000000000 ) ) ;
#4306=CARTESIAN_POINT ( 'NONE',  ( -28.68588794268873698, -129.7637193493918915, 0.000000000000000000 ) ) ;
#4309=EDGE_CURVE ( 'NONE', #4929, #11681, #1275, .T. ) ;
#4314=EDGE_LOOP ( 'NONE', ( #16670, #13987, #14510, #12809 ) ) ;
#4320=ORIENTED_EDGE ( 'NONE', *, *, #20004, .T. ) ;
#4331=PLANE ( 'NONE',  #5548 ) ;
#4332=EDGE_CURVE ( 'NONE', #15817, #11167, #19437, .T. ) ;
#4337=ORIENTED_EDGE ( 'NONE', *, *, #6785, .F. ) ;
#4339=VERTEX_POINT ( 'NONE', #16635 ) ;
#4343=CARTESIAN_POINT ( 'NONE',  ( 60.03793209889851568, 10.52886280891152104, 131.1729372809869005 ) ) ;
#4355=CARTESIAN_POINT ( 'NONE',  ( 20.42502041961813219, 290.7078131342035476, -7.833137205859951102 ) ) ;
#4356=LINE ( 'NONE', #20694, #12994 ) ;
#4362=VECTOR ( 'NONE', #1875, 1000.000000000000114 ) ;
#4363=VERTEX_POINT ( 'NONE', #1709 ) ;
#4367=AXIS2_PLACEMENT_3D ( 'NONE', #19101, #20724, #18658 ) ;
#4372=ORIENTED_EDGE ( 'NONE', *, *, #15849, .F. ) ;
#4374=CYLINDRICAL_SURFACE ( 'NONE', #9640, 4.000000000000001776 ) ;
#4376=DIRECTION ( 'NONE',  ( 0.000000000000000000, -1.000000000000000000, 0.000000000000000000 ) ) ;
#4377=LINE ( 'NONE', #20827, #2671 ) ;
#4378=LINE ( 'NONE', #20605, #6332 ) ;
#4388=DIRECTION ( 'NONE',  ( 0.000000000000000000, 0.000000000000000000, 1.000000000000000000 ) ) ;
#4398=VERTEX_POINT ( 'NONE', #6550 ) ;
#4404=ADVANCED_FACE ( 'NONE', ( #18347 ), #11538, .F. ) ;
#4407=PRODUCT ( 'Heavy Arch Steel Frame Casting', 'Heavy Arch Steel Frame Casting', '', ( #18096 ) ) ;
#4409=CARTESIAN_POINT ( 'NONE',  ( 40.42502041961814996, 180.1716627696692967, 20.00000000000000355 ) ) ;
#4417=ADVANCED_FACE ( 'NONE', ( #10122 ), #15222, .F. ) ;
#4426=ORIENTED_EDGE ( 'NONE', *, *, #3235, .F. ) ;
#4427=EDGE_CURVE ( 'NONE', #15324, #604, #15123, .T. ) ;
#4435=CARTESIAN_POINT ( 'NONE',  ( 77.07016797226398808, 161.6844911138030056, 40.00000000000000000 ) ) ;
#4437=PLANE ( 'NONE',  #4937 ) ;
#4442=VERTEX_POINT ( 'NONE', #6874 ) ;
#4444=ORIENTED_EDGE ( 'NONE', *, *, #13069, .F. ) ;
#4445=CARTESIAN_POINT ( 'NONE',  ( -28.68588794268872988, 10.52886280891152104, -49.60091809715359545 ) ) ;
#4462=CARTESIAN_POINT ( 'NONE',  ( 0.000000000000000000, 30.52886280891154058, 0.000000000000000000 ) ) ;
#4463=CARTESIAN_POINT ( 'NONE',  ( 52.60622592008805043, 30.52886280891152282, 151.0302712373927250 ) ) ;
#4468=EDGE_CURVE ( 'NONE', #983, #554, #8710, .T. ) ;
#4475=ORIENTED_EDGE ( 'NONE', *, *, #11277, .T. ) ;
#4479=DIRECTION ( 'NONE',  ( -1.000000000000000000, 0.000000000000000000, 0.000000000000000000 ) ) ;
#4483=DIRECTION ( 'NONE',  ( -0.000000000000000000, 1.000000000000000000, -0.000000000000000000 ) ) ;
#4486=FACE_OUTER_BOUND ( 'NONE', #1336, .T. ) ;
#4490=VECTOR ( 'NONE', #9418, 1000.000000000000000 ) ;
#4493=CARTESIAN_POINT ( 'NONE',  ( 71.32175588950862277, 75.31183677523708297, -94.99999999999994316 ) ) ;
#4498=CARTESIAN_POINT ( 'NONE',  ( -49.57497958038185715, 160.1716627696692683, -60.00000000000000000 ) ) ;
#4509=FACE_OUTER_BOUND ( 'NONE', #1394, .T. ) ;
#4510=AXIS2_PLACEMENT_3D ( 'NONE', #851, #5908, #17483 ) ;
#4512=DIRECTION ( 'NONE',  ( -1.000000000000000000, -0.000000000000000000, 0.000000000000000000 ) ) ;
#4515=FACE_OUTER_BOUND ( 'NONE', #9042, .T. ) ;
#4520=CARTESIAN_POINT ( 'NONE',  ( 0.000000000000000000, -343.0245277843623057, 0.000000000000000000 ) ) ;
#4523=VECTOR ( 'NONE', #12179, 1000.000000000000114 ) ;
#4540=CARTESIAN_POINT ( 'NONE',  ( 52.60622592008805043, 10.52886280891152104, 151.0302712373927250 ) ) ;
#4546=EDGE_CURVE ( 'NONE', #19853, #5504, #15755, .T. ) ;
#4548=FACE_OUTER_BOUND ( 'NONE', #6531, .T. ) ;
#4549=EDGE_LOOP ( 'NONE', ( #1804, #11307, #4815, #14469 ) ) ;
#4551=VERTEX_POINT ( 'NONE', #9246 ) ;
#4554=AXIS2_PLACEMENT_3D ( 'NONE', #19903, #10051, #19477 ) ;
#4556=LINE ( 'NONE', #2835, #4490 ) ;
#4557=VECTOR ( 'NONE', #15783, 999.9999999999998863 ) ;
#4559=DIRECTION ( 'NONE',  ( 1.000000000000000000, 0.000000000000000000, 0.000000000000000000 ) ) ;
#4565=CARTESIAN_POINT ( 'NONE',  ( 105.7989814974898479, 142.5259582928263455, 20.00000000000000355 ) ) ;
#4569=LINE ( 'NONE', #1127, #14559 ) ;
#4570=LINE ( 'NONE', #17446, #20607 ) ;
#4579=AXIS2_PLACEMENT_3D ( 'NONE', #8036, #10967, #17575 ) ;
#4580=DIRECTION ( 'NONE',  ( -1.232945044042657126E-32, 9.855701800883825964E-17, 1.000000000000000000 ) ) ;
#4584=VERTEX_POINT ( 'NONE', #12065 ) ;
#4586=CARTESIAN_POINT ( 'NONE',  ( 35.96497763894179656, 170.1716627696692683, 57.37501161332323107 ) ) ;
#4589=FACE_OUTER_BOUND ( 'NONE', #1990, .T. ) ;
#4594=FACE_OUTER_BOUND ( 'NONE', #15211, .T. ) ;
#4599=FACE_BOUND ( 'NONE', #6370, .T. ) ;
#4602=ORIENTED_EDGE ( 'NONE', *, *, #3842, .T. ) ;
#4603=ORIENTED_EDGE ( 'NONE', *, *, #19059, .F. ) ;
#4604=FACE_OUTER_BOUND ( 'NONE', #3799, .T. ) ;
#4608=CIRCLE ( 'NONE', #16715, 43.46661168214937732 ) ;
#4610=CARTESIAN_POINT ( 'NONE',  ( 29.72350413846044859, 280.4463447002762564, -20.00000000000000355 ) ) ;
#4614=DIRECTION ( 'NONE',  ( 0.000000000000000000, 0.000000000000000000, -1.000000000000000000 ) ) ;
#4620=CARTESIAN_POINT ( 'NONE',  ( 80.02941346738570871, 139.7547175612648402, 70.25248122596298117 ) ) ;
#4623=AXIS2_PLACEMENT_3D ( 'NONE', #18751, #4580, #12804 ) ;
#4626=CIRCLE ( 'NONE', #7381, 49.60091809715359545 ) ;
#4640=VECTOR ( 'NONE', #8021, 1000.000000000000000 ) ;
#4643=CARTESIAN_POINT ( 'NONE',  ( 28.16023193154655502, 323.8848358243226357, -20.00000000000000355 ) ) ;
#4647=CARTESIAN_POINT ( 'NONE',  ( -18.68588794268873698, 281.1055109169419666, 20.00000000000000355 ) ) ;
#4649=DIRECTION ( 'NONE',  ( 0.000000000000000000, -1.000000000000000000, 0.000000000000000000 ) ) ;
#4651=DIRECTION ( 'NONE',  ( 0.000000000000000000, 0.000000000000000000, 1.000000000000000000 ) ) ;
#4652=EDGE_LOOP ( 'NONE', ( #2597, #16221, #7909, #17273, #13763 ) ) ;
#4678=ORIENTED_EDGE ( 'NONE', *, *, #1355, .F. ) ;
#4681=CARTESIAN_POINT ( 'NONE',  ( -18.68588794268873698, 281.1055109169419666, -20.00000000000000355 ) ) ;
#4687=CARTESIAN_POINT ( 'NONE',  ( 0.000000000000000000, 31.85652257517428865, 0.000000000000000000 ) ) ;
#4690=CARTESIAN_POINT ( 'NONE',  ( -23.30554231582819469, 45.34767784731757700, 49.31100188924479966 ) ) ;
#4693=DIRECTION ( 'NONE',  ( 0.000000000000000000, -1.000000000000000000, 0.000000000000000000 ) ) ;
#4699=CARTESIAN_POINT ( 'NONE',  ( 30.42502041961813575, 271.1055109169419097, -20.00000000000000355 ) ) ;
#4700=B_SPLINE_CURVE_WITH_KNOTS ( 'NONE', 3,
 ( #15113, #10114, #8490, #85, #6651, #8383, #5147, #15007, #8704, #10214, #11636, #5456, #297, #18231, #19858, #5035, #15326, #18646, #3423, #6866, #19968, #193, #10002, #18545, #13378, #20078, #12058, #20286, #3838, #16625, #1700, #16735, #11745, #1922, #11850, #11951, #18446, #3632, #16837, #407 ),
 .UNSPECIFIED., .F., .F.,
 ( 4, 2, 2, 2, 2, 2, 2, 2, 2, 2, 2, 2, 2, 2, 2, 2, 2, 2, 2, 4 ),
 ( 0.000000000000000000, 0.003131370304449435787, 0.004697055456674143273, 0.006262740608898849023, 0.007045583185011209705, 0.007828425761123570387, 0.009394110913348300423, 0.01095979606557302699, 0.01174263864168539201, 0.01252548121779775703, 0.01409116637002248706, 0.01487400894613485382, 0.01565685152224722057, 0.01878822182669671534, 0.01957106440280908730, 0.02035390697892145925, 0.02191959213114619623, 0.02270243470725856819, 0.02348527728337093667, 0.02505096243559567018 ),
 .UNSPECIFIED. ) ;
#4712=LINE ( 'NONE', #11309, #20013 ) ;
#4720=CARTESIAN_POINT ( 'NONE',  ( 20.42502041961813575, 271.1055109169419666, -40.00000000000000000 ) ) ;
#4721=EDGE_CURVE ( 'NONE', #2882, #983, #14671, .T. ) ;
#4723=DIRECTION ( 'NONE',  ( 0.000000000000000000, -0.000000000000000000, -1.000000000000000000 ) ) ;
#4731=VECTOR ( 'NONE', #15835, 1000.000000000000000 ) ;
#4735=DIRECTION ( 'NONE',  ( 0.000000000000000000, -1.000000000000000000, 0.000000000000000000 ) ) ;
#4746=CARTESIAN_POINT ( 'NONE',  ( -162.2727221670389781, 30.52886280891152282, -20.57735571454641033 ) ) ;
#4751=FACE_OUTER_BOUND ( 'NONE', #7459, .T. ) ;
#4752=ORIENTED_EDGE ( 'NONE', *, *, #1121, .T. ) ;
#4756=ORIENTED_EDGE ( 'NONE', *, *, #21293, .T. ) ;
#4761=EDGE_CURVE ( 'NONE', #14968, #17590, #19306, .T. ) ;
#4780=DIRECTION ( 'NONE',  ( 0.000000000000000000, 0.000000000000000000, -1.000000000000000000 ) ) ;
#4792=CARTESIAN_POINT ( 'NONE',  ( -10.76731745429010090, 56.85652257517428865, 46.25122601329427141 ) ) ;
#4795=DIRECTION ( 'NONE',  ( -0.000000000000000000, -0.000000000000000000, 1.000000000000000000 ) ) ;
#4799=DIRECTION ( 'NONE',  ( 1.000000000000000000, 0.000000000000000000, 2.399110633850889130E-16 ) ) ;
#4806=ORIENTED_EDGE ( 'NONE', *, *, #11450, .T. ) ;
#4812=ORIENTED_EDGE ( 'NONE', *, *, #21337, .F. ) ;
#4815=ORIENTED_EDGE ( 'NONE', *, *, #11157, .T. ) ;
#4820=CARTESIAN_POINT ( 'NONE',  ( 60.03793209889851568, 10.52886280891152104, -131.1729372809869005 ) ) ;
#4824=CARTESIAN_POINT ( 'NONE',  ( 0.000000000000000000, 0.000000000000000000, -40.00000000000000000 ) ) ;
#4834=DIRECTION ( 'NONE',  ( 0.000000000000000000, 1.000000000000000000, 0.000000000000000000 ) ) ;
#4837=DIRECTION ( 'NONE',  ( 0.000000000000000000, 0.000000000000000000, 1.000000000000000000 ) ) ;
#4840=ORIENTED_EDGE ( 'NONE', *, *, #3638, .F. ) ;
#4843=EDGE_CURVE ( 'NONE', #7864, #16350, #20058, .T. ) ;
#4847=LINE ( 'NONE', #17626, #6463 ) ;
#4848=EDGE_CURVE ( 'NONE', #12430, #14255, #11832, .T. ) ;
#4850=EDGE_CURVE ( 'NONE', #4363, #16962, #16500, .T. ) ;
#4851=FACE_OUTER_BOUND ( 'NONE', #17407, .T. ) ;
#4852=VECTOR ( 'NONE', #19216, 1000.000000000000000 ) ;
#4853=AXIS2_PLACEMENT_3D ( 'NONE', #19384, #19178, #2954 ) ;
#4855=VECTOR ( 'NONE', #5854, 1000.000000000000000 ) ;
#4868=DIRECTION ( 'NONE',  ( 1.000000000000000000, 0.000000000000000000, 0.000000000000000000 ) ) ;
#4870=CARTESIAN_POINT ( 'NONE',  ( 51.93385628276429600, 30.52886280891152282, -94.99999999999994316 ) ) ;
#4872=VECTOR ( 'NONE', #4799, 1000.000000000000000 ) ;
#4880=CARTESIAN_POINT ( 'NONE',  ( 91.21585410611801592, 31.85652257517428865, 40.00000000000000000 ) ) ;
#4882=CARTESIAN_POINT ( 'NONE',  ( -33.45347746554494961, 53.84009227044784041, 120.4403519833905136 ) ) ;
#4883=LINE ( 'NONE', #9846, #14902 ) ;
#4894=ORIENTED_EDGE ( 'NONE', *, *, #19094, .T. ) ;
#4895=CARTESIAN_POINT ( 'NONE',  ( -33.84809828339280102, 56.85652257517428865, -120.3299889578561448 ) ) ;
#4899=CARTESIAN_POINT ( 'NONE',  ( -18.68588794268873698, 323.8848358243226357, 20.00000000000000355 ) ) ;
#4904=DIRECTION ( 'NONE',  ( 0.000000000000000000, -1.000000000000000000, 0.000000000000000000 ) ) ;
#4907=CYLINDRICAL_SURFACE ( 'NONE', #12688, 10.00000000000000178 ) ;
#4908=CARTESIAN_POINT ( 'NONE',  ( 60.03793209889851568, 30.52886280891152282, -131.1729372809869005 ) ) ;
#4914=B_SPLINE_CURVE_WITH_KNOTS ( 'NONE', 3,
 ( #3429, #10009, #15015, #9756, #11170, #6508, #6729, #6298, #9970, #13126, #6616, #16380, #13013, #19711 ),
 .UNSPECIFIED., .F., .F.,
 ( 4, 2, 2, 2, 2, 2, 4 ),
 ( 0.000000000000000000, 0.002830465529762977734, 0.004245698294644466818, 0.005660931059525955468, 0.007076163824407444118, 0.008491396589288933636, 0.01132186211905188838 ),
 .UNSPECIFIED. ) ;
#4921=CARTESIAN_POINT ( 'NONE',  ( 77.07016797226398808, 161.6844911138030056, -40.00000000000000000 ) ) ;
#4922=ORIENTED_EDGE ( 'NONE', *, *, #19987, .F. ) ;
#4929=VERTEX_POINT ( 'NONE', #5438 ) ;
#4935=CARTESIAN_POINT ( 'NONE',  ( 81.24038404635965094, 30.52886280891152282, 131.1729372809869005 ) ) ;
#4936=CARTESIAN_POINT ( 'NONE',  ( 125.7989814974898053, 10.52886280891152104, 40.00000000000000000 ) ) ;
#4937=AXIS2_PLACEMENT_3D ( 'NONE', #14083, #17425, #2501 ) ;
#4944=CARTESIAN_POINT ( 'NONE',  ( -15.54750367907772635, 45.31613216062294214, -120.2864949470673110 ) ) ;
#4948=VECTOR ( 'NONE', #18651, 1000.000000000000000 ) ;
#4950=ADVANCED_FACE ( 'NONE', ( #17341 ), #7479, .F. ) ;
#4953=( NAMED_UNIT ( * ) SI_UNIT ( $, .STERADIAN. ) SOLID_ANGLE_UNIT ( ) );
#4959=AXIS2_PLACEMENT_3D ( 'NONE', #13611, #8720, #15133 ) ;
#4966=CARTESIAN_POINT ( 'NONE',  ( -28.68588794268872988, -129.7637193493918915, -49.60091809715359545 ) ) ;
#4982=CARTESIAN_POINT ( 'NONE',  ( 62.02695467647412642, 160.1716627696692399, -61.71700053422263466 ) ) ;
#4985=CARTESIAN_POINT ( 'NONE',  ( 40.42502041961814996, 180.1716627696692967, -20.00000000000000355 ) ) ;
#4987=LINE ( 'NONE', #18393, #21195 ) ;
#4990=EDGE_CURVE ( 'NONE', #15032, #14472, #17028, .T. ) ;
#4991=LINE ( 'NONE', #6495, #6813 ) ;
#4994=CARTESIAN_POINT ( 'NONE',  ( 35.96497763894178945, 230.5765313837437418, -60.00000000000000000 ) ) ;
#5000=ORIENTED_EDGE ( 'NONE', *, *, #17107, .T. ) ;
#5002=ORIENTED_EDGE ( 'NONE', *, *, #11425, .T. ) ;
#5005=CARTESIAN_POINT ( 'NONE',  ( 51.98438129372387806, 30.52886280891151216, 117.7249735956185219 ) ) ;
#5010=CARTESIAN_POINT ( 'NONE',  ( 52.60622592008805043, 10.52886280891152104, -151.0302712373927250 ) ) ;
#5012=CARTESIAN_POINT ( 'NONE',  ( -18.70553453894068952, 45.88067589482868414, 48.58894481687972444 ) ) ;
#5025=VERTEX_POINT ( 'NONE', #15411 ) ;
#5035=CARTESIAN_POINT ( 'NONE',  ( -15.73313710990876402, 47.36853976159893165, -47.88030834489089926 ) ) ;
#5039=CARTESIAN_POINT ( 'NONE',  ( 40.42502041961814996, 180.1716627696692967, 40.00000000000000000 ) ) ;
#5040=CARTESIAN_POINT ( 'NONE',  ( 65.85920792673738333, 160.1716627696692683, -40.00000000000000000 ) ) ;
#5041=FACE_OUTER_BOUND ( 'NONE', #3827, .T. ) ;
#5048=CYLINDRICAL_SURFACE ( 'NONE', #8523, 10.00000000000000178 ) ;
#5051=EDGE_CURVE ( 'NONE', #5934, #15977, #13892, .T. ) ;
#5053=CARTESIAN_POINT ( 'NONE',  ( -10.76731745429009912, 56.85652257517428865, 118.3724535612433186 ) ) ;
#5063=LINE ( 'NONE', #14927, #6543 ) ;
#5065=DIRECTION ( 'NONE',  ( 0.000000000000000000, 0.000000000000000000, 1.000000000000000000 ) ) ;
#5072=VECTOR ( 'NONE', #1570, 1000.000000000000000 ) ;
#5075=ORIENTED_EDGE ( 'NONE', *, *, #1422, .F. ) ;
#5078=ORIENTED_EDGE ( 'NONE', *, *, #20990, .T. ) ;
#5090=VECTOR ( 'NONE', #2953, 1000.000000000000000 ) ;
#5092=FACE_OUTER_BOUND ( 'NONE', #10821, .T. ) ;
#5094=FACE_OUTER_BOUND ( 'NONE', #5448, .T. ) ;
#5097=DIRECTION ( 'NONE',  ( -0.000000000000000000, -0.000000000000000000, -1.000000000000000000 ) ) ;
#5103=VERTEX_POINT ( 'NONE', #9002 ) ;
#5108=VERTEX_POINT ( 'NONE', #5754 ) ;
#5109=DIRECTION ( 'NONE',  ( 0.000000000000000000, 1.000000000000000000, 0.000000000000000000 ) ) ;
#5125=EDGE_CURVE ( 'NONE', #17724, #2963, #4569, .T. ) ;
#5126=CARTESIAN_POINT ( 'NONE',  ( -162.2727221670389781, 10.52886280891152104, 20.57735571454641033 ) ) ;
#5129=EDGE_CURVE ( 'NONE', #16429, #15603, #15940, .T. ) ;
#5136=ORIENTED_EDGE ( 'NONE', *, *, #19094, .F. ) ;
#5138=ORIENTED_EDGE ( 'NONE', *, *, #10446, .T. ) ;
#5142=ORIENTED_EDGE ( 'NONE', *, *, #15447, .F. ) ;
#5147=CARTESIAN_POINT ( 'NONE',  ( -12.15536544594166557, 51.34507591104713953, -46.76614217995071954 ) ) ;
#5149=DIRECTION ( 'NONE',  ( -0.000000000000000000, -0.000000000000000000, -1.000000000000000000 ) ) ;
#5150=CARTESIAN_POINT ( 'NONE',  ( -18.68588794268873698, 281.1055109169419666, -20.00000000000000355 ) ) ;
#5152=DIRECTION ( 'NONE',  ( 1.000000000000000000, -0.000000000000000000, 0.000000000000000000 ) ) ;
#5153=DIRECTION ( 'NONE',  ( 1.000000000000000000, -0.000000000000000000, -0.000000000000000000 ) ) ;
#5160=CARTESIAN_POINT ( 'NONE',  ( 88.28695088269886071, 152.5259582928263740, 20.00000000000000355 ) ) ;
#5162=ORIENTED_EDGE ( 'NONE', *, *, #300, .F. ) ;
#5163=LINE ( 'NONE', #16752, #11180 ) ;
#5174=DIRECTION ( 'NONE',  ( -0.000000000000000000, -1.000000000000000000, -0.000000000000000000 ) ) ;
#5178=EDGE_CURVE ( 'NONE', #20702, #15032, #10839, .T. ) ;
#5183=ORIENTED_EDGE ( 'NONE', *, *, #16038, .F. ) ;
#5184=AXIS2_PLACEMENT_3D ( 'NONE', #1348, #7921, #21135 ) ;
#5225=FACE_OUTER_BOUND ( 'NONE', #10918, .T. ) ;
#5230=LINE ( 'NONE', #3505, #8285 ) ;
#5247=EDGE_CURVE ( 'NONE', #7551, #9807, #19708, .T. ) ;
#5248=AXIS2_PLACEMENT_3D ( 'NONE', #16418, #10994, #3110 ) ;
#5253=CARTESIAN_POINT ( 'NONE',  ( 65.85920792673738333, 160.1716627696692683, -40.00000000000000000 ) ) ;
#5254=DIRECTION ( 'NONE',  ( 0.000000000000000000, 0.000000000000000000, -1.000000000000000000 ) ) ;
#5260=EDGE_CURVE ( 'NONE', #454, #4584, #18341, .T. ) ;
#5275=CARTESIAN_POINT ( 'NONE',  ( 105.7989814974898479, 142.5259582928263455, 40.00000000000000000 ) ) ;
#5276=CYLINDRICAL_SURFACE ( 'NONE', #4232, 9.999999999999994671 ) ;
#5277=AXIS2_PLACEMENT_3D ( 'NONE', #20158, #5326, #10086 ) ;
#5288=VERTEX_POINT ( 'NONE', #14641 ) ;
#5296=VECTOR ( 'NONE', #9079, 1000.000000000000000 ) ;
#5299=DIRECTION ( 'NONE',  ( -0.000000000000000000, -0.000000000000000000, -1.000000000000000000 ) ) ;
#5315=ORIENTED_EDGE ( 'NONE', *, *, #18995, .T. ) ;
#5321=DIRECTION ( 'NONE',  ( -0.000000000000000000, -0.000000000000000000, -1.000000000000000000 ) ) ;
#5326=DIRECTION ( 'NONE',  ( 0.000000000000000000, 1.000000000000000000, 0.000000000000000000 ) ) ;
#5334=PLANE ( 'NONE',  #14404 ) ;
#5337=DIRECTION ( 'NONE',  ( 1.000000000000000000, 0.000000000000000000, 0.000000000000000000 ) ) ;
#5345=ORIENTED_EDGE ( 'NONE', *, *, #4201, .T. ) ;
#5353=CYLINDRICAL_SURFACE ( 'NONE', #14088, 5.000000000000004441 ) ;
#5355=CARTESIAN_POINT ( 'NONE',  ( 82.89408817951444064, 286.0648460576640559, -40.00000000000000000 ) ) ;
#5356=CARTESIAN_POINT ( 'NONE',  ( 115.7989814974898337, 142.5259582928263455, 40.00000000000000000 ) ) ;
#5361=CARTESIAN_POINT ( 'NONE',  ( -32.02117626164387332, 50.55271151534634555, -49.49072515476203904 ) ) ;
#5366=ORIENTED_EDGE ( 'NONE', *, *, #2802, .F. ) ;
#5370=EDGE_CURVE ( 'NONE', #17507, #16345, #4883, .T. ) ;
#5371=EDGE_LOOP ( 'NONE', ( #11785, #18087, #14338, #16329, #16409, #8454, #9476, #16984, #17255, #16905, #15469, #19552, #18190, #5002, #772, #5607, #7678, #8260, #6858, #20036, #4894, #14599, #1474, #20974, #8831, #11872 ) ) ;
#5382=EDGE_CURVE ( 'NONE', #12221, #5798, #8113, .T. ) ;
#5387=VECTOR ( 'NONE', #948, 1000.000000000000000 ) ;
#5388=ORIENTED_EDGE ( 'NONE', *, *, #6057, .F. ) ;
#5391=EDGE_LOOP ( 'NONE', ( #7843, #5609 ) ) ;
#5395=( BOUNDED_CURVE ( )  B_SPLINE_CURVE ( 3, ( #2440, #7501, #12279, #2650 ),
 .UNSPECIFIED., .F., .T. ) 
 B_SPLINE_CURVE_WITH_KNOTS ( ( 4, 4 ),
 ( 4.712388980384689674, 6.260350157286452166 ),
 .UNSPECIFIED. ) 
 CURVE ( )  GEOMETRIC_REPRESENTATION_ITEM ( )  RATIONAL_B_SPLINE_CURVE ( ( 1.000000000000000000, 0.8100893075783979214, 0.8100893075783979214, 1.000000000000000000 ) ) 
 REPRESENTATION_ITEM ( '' )  );
#5401=VECTOR ( 'NONE', #19415, 1000.000000000000000 ) ;
#5410=LINE ( 'NONE', #2289, #14633 ) ;
#5417=ORIENTED_EDGE ( 'NONE', *, *, #2481, .T. ) ;
#5426=CARTESIAN_POINT ( 'NONE',  ( 71.32175588950862277, 75.31183677523708297, 94.99999999999994316 ) ) ;
#5438=CARTESIAN_POINT ( 'NONE',  ( -49.57497958038185715, 160.1716627696692683, -60.00000000000000000 ) ) ;
#5440=EDGE_CURVE ( 'NONE', #16962, #14726, #15171, .T. ) ;
#5441=VECTOR ( 'NONE', #5492, 1000.000000000000000 ) ;
#5448=EDGE_LOOP ( 'NONE', ( #20546, #1445, #35, #8556, #6297, #18543, #15558, #632, #17197, #21209, #8185, #12544 ) ) ;
#5450=CARTESIAN_POINT ( 'NONE',  ( 28.16023193154655502, 323.8848358243226357, -20.00000000000000355 ) ) ;
#5452=DIRECTION ( 'NONE',  ( 0.000000000000000000, -1.000000000000000000, 0.000000000000000000 ) ) ;
#5454=VERTEX_POINT ( 'NONE', #16471 ) ;
#5456=CARTESIAN_POINT ( 'NONE',  ( -13.63080313027055901, 49.23037255044063443, -47.26215086388379660 ) ) ;
#5457=EDGE_CURVE ( 'NONE', #11304, #1316, #19019, .T. ) ;
#5459=DIRECTION ( 'NONE',  ( 0.000000000000000000, -1.000000000000000000, 0.000000000000000000 ) ) ;
#5462=CARTESIAN_POINT ( 'NONE',  ( 35.96497763894178945, 230.5765313837437418, 60.00000000000000000 ) ) ;
#5472=DIRECTION ( 'NONE',  ( -1.000000000000000000, 0.000000000000000000, 0.000000000000000000 ) ) ;
#5477=ORIENTED_EDGE ( 'NONE', *, *, #16647, .T. ) ;
#5483=VECTOR ( 'NONE', #7179, 1000.000000000000114 ) ;
#5492=DIRECTION ( 'NONE',  ( -1.000000000000000000, 0.000000000000000000, 0.000000000000000000 ) ) ;
#5497=VERTEX_POINT ( 'NONE', #15599 ) ;
#5504=VERTEX_POINT ( 'NONE', #15385 ) ;
#5519=DIRECTION ( 'NONE',  ( -0.000000000000000000, -0.000000000000000000, -1.000000000000000000 ) ) ;
#5521=EDGE_CURVE ( 'NONE', #15324, #10233, #392, .T. ) ;
#5533=VECTOR ( 'NONE', #10449, 1000.000000000000114 ) ;
#5540=LINE ( 'NONE', #588, #10324 ) ;
#5544=CARTESIAN_POINT ( 'NONE',  ( 19.47671684378140355, 160.1716627696692683, -61.31874706328063240 ) ) ;
#5548=AXIS2_PLACEMENT_3D ( 'NONE', #4647, #4228, #2606 ) ;
#5549=CARTESIAN_POINT ( 'NONE',  ( -33.46524870589303902, 53.80964298180775529, -120.4371303356476091 ) ) ;
#5552=VERTEX_POINT ( 'NONE', #17424 ) ;
#5559=DIRECTION ( 'NONE',  ( 0.000000000000000000, -1.000000000000000000, 0.000000000000000000 ) ) ;
#5562=VERTEX_POINT ( 'NONE', #20986 ) ;
#5564=CARTESIAN_POINT ( 'NONE',  ( 6.416697501590670427, 172.9933428177121471, 45.00000000000000000 ) ) ;
#5574=ADVANCED_FACE ( 'NONE', ( #19157 ), #4331, .F. ) ;
#5575=CARTESIAN_POINT ( 'NONE',  ( -49.57497958038186425, 230.5765313837437418, 60.00000000000000000 ) ) ;
#5584=VECTOR ( 'NONE', #21183, 1000.000000000000000 ) ;
#5595=FACE_OUTER_BOUND ( 'NONE', #11007, .T. ) ;
#5607=ORIENTED_EDGE ( 'NONE', *, *, #9290, .T. ) ;
#5609=ORIENTED_EDGE ( 'NONE', *, *, #7649, .F. ) ;
#5610=EDGE_LOOP ( 'NONE', ( #13683, #14889, #1365, #9706, #12452, #12724 ) ) ;
#5647=EDGE_CURVE ( 'NONE', #2506, #14726, #2928, .T. ) ;
#5649=CARTESIAN_POINT ( 'NONE',  ( 29.72350413846044859, 280.4463447002762564, 40.00000000000000000 ) ) ;
#5655=DIRECTION ( 'NONE',  ( 0.4989387216749511800, 0.8666372666885294729, 0.000000000000000000 ) ) ;
#5658=CARTESIAN_POINT ( 'NONE',  ( -29.89242224052212293, 48.12632300629133653, -121.3744031878869976 ) ) ;
#5664=CARTESIAN_POINT ( 'NONE',  ( 78.68120802659204571, 149.7457237375499517, 20.00000000000000355 ) ) ;
#5678=CARTESIAN_POINT ( 'NONE',  ( 81.24038404635966515, 10.52886280891152104, -94.99999999999994316 ) ) ;
#5687=ORIENTED_EDGE ( 'NONE', *, *, #20422, .F. ) ;
#5688=ORIENTED_EDGE ( 'NONE', *, *, #14401, .T. ) ;
#5690=ORIENTED_EDGE ( 'NONE', *, *, #9426, .F. ) ;
#5698=DIRECTION ( 'NONE',  ( 1.000000000000000000, 1.250996701150283068E-16, -0.000000000000000000 ) ) ;
#5699=VECTOR ( 'NONE', #18581, 1000.000000000000000 ) ;
#5710=ORIENTED_EDGE ( 'NONE', *, *, #14743, .T. ) ;
#5712=VERTEX_POINT ( 'NONE', #5945 ) ;
#5713=ORIENTED_EDGE ( 'NONE', *, *, #5129, .T. ) ;
#5715=CARTESIAN_POINT ( 'NONE',  ( 6.416697501590670427, 217.7548513357008630, 60.00000000000000000 ) ) ;
#5718=EDGE_LOOP ( 'NONE', ( #10263, #16298, #15111, #6585, #10764, #20245, #5688, #17006, #15049, #1552, #10951, #12239, #18301, #16188, #4756, #3569, #14815 ) ) ;
#5729=DIRECTION ( 'NONE',  ( 0.000000000000000000, 0.000000000000000000, -1.000000000000000000 ) ) ;
#5736=ORIENTED_EDGE ( 'NONE', *, *, #3454, .F. ) ;
#5742=CARTESIAN_POINT ( 'NONE',  ( 88.28695088269886071, 142.5259582928263455, 20.00000000000000355 ) ) ;
#5750=DIRECTION ( 'NONE',  ( 0.000000000000000000, 0.000000000000000000, 1.000000000000000000 ) ) ;
#5753=CARTESIAN_POINT ( 'NONE',  ( 20.42502041961814641, 160.1716627696692683, 40.00000000000000000 ) ) ;
#5754=CARTESIAN_POINT ( 'NONE',  ( 27.98965548446208729, 333.8848358243226357, -40.00000000000000000 ) ) ;
#5758=CARTESIAN_POINT ( 'NONE',  ( -31.43925259815332041, 49.75942336920967790, -120.9825033997044557 ) ) ;
#5761=VECTOR ( 'NONE', #15622, 1000.000000000000000 ) ;
#5765=ORIENTED_EDGE ( 'NONE', *, *, #17085, .F. ) ;
#5776=VECTOR ( 'NONE', #8163, 1000.000000000000000 ) ;
#5778=DIRECTION ( 'NONE',  ( 1.000000000000000000, 0.000000000000000000, 0.000000000000000000 ) ) ;
#5783=EDGE_CURVE ( 'NONE', #19677, #14197, #1205, .T. ) ;
#5784=CIRCLE ( 'NONE', #13033, 9.999999999999994671 ) ;
#5785=DIRECTION ( 'NONE',  ( 1.000000000000000000, 0.000000000000000000, 0.000000000000000000 ) ) ;
#5798=VERTEX_POINT ( 'NONE', #18050 ) ;
#5802=CARTESIAN_POINT ( 'NONE',  ( 51.50493485826542184, 170.1716627696692683, -57.52045949366692668 ) ) ;
#5806=LINE ( 'NONE', #858, #7723 ) ;
#5809=CARTESIAN_POINT ( 'NONE',  ( 35.96497763894178945, 170.1716627696692683, 40.00000000000000000 ) ) ;
#5817=VECTOR ( 'NONE', #19223, 1000.000000000000000 ) ;
#5818=DIRECTION ( 'NONE',  ( 1.000000000000000000, 0.000000000000000000, 0.000000000000000000 ) ) ;
#5820=ORIENTED_EDGE ( 'NONE', *, *, #6980, .F. ) ;
#5822=DIRECTION ( 'NONE',  ( 1.000000000000000000, 0.000000000000000000, 0.000000000000000000 ) ) ;
#5823=ORIENTED_EDGE ( 'NONE', *, *, #7414, .F. ) ;
#5842=ORIENTED_EDGE ( 'NONE', *, *, #5178, .T. ) ;
#5845=EDGE_LOOP ( 'NONE', ( #14172, #9672, #9254, #6479 ) ) ;
#5847=ORIENTED_EDGE ( 'NONE', *, *, #18947, .F. ) ;
#5854=DIRECTION ( 'NONE',  ( -0.9365583756827543516, 0.000000000000000000, -0.3505116388060184329 ) ) ;
#5876=VECTOR ( 'NONE', #17356, 1000.000000000000000 ) ;
#5880=DIRECTION ( 'NONE',  ( 0.000000000000000000, 0.000000000000000000, 1.000000000000000000 ) ) ;
#5882=EDGE_LOOP ( 'NONE', ( #15235, #6803, #2672, #14602 ) ) ;
#5892=CIRCLE ( 'NONE', #17973, 5.000000000000004441 ) ;
#5902=ORIENTED_EDGE ( 'NONE', *, *, #5247, .T. ) ;
#5905=ORIENTED_EDGE ( 'NONE', *, *, #18034, .F. ) ;
#5908=DIRECTION ( 'NONE',  ( 0.000000000000000000, 0.000000000000000000, 1.000000000000000000 ) ) ;
#5912=LINE ( 'NONE', #16089, #12810 ) ;
#5914=CARTESIAN_POINT ( 'NONE',  ( 20.42502041961813575, 271.1055109169419666, -20.00000000000000355 ) ) ;
#5923=FACE_OUTER_BOUND ( 'NONE', #15443, .T. ) ;
#5925=AXIS2_PLACEMENT_3D ( 'NONE', #9498, #13073, #21284 ) ;
#5929=DIRECTION ( 'NONE',  ( 0.000000000000000000, -1.000000000000000000, 0.000000000000000000 ) ) ;
#5934=VERTEX_POINT ( 'NONE', #11344 ) ;
#5945=CARTESIAN_POINT ( 'NONE',  ( 91.21585410611801592, 31.85652257517428865, -85.46735025547123143 ) ) ;
#5960=EDGE_CURVE ( 'NONE', #4339, #14946, #5892, .T. ) ;
#5982=EDGE_CURVE ( 'NONE', #13870, #264, #6690, .T. ) ;
#5983=ORIENTED_EDGE ( 'NONE', *, *, #11593, .T. ) ;
#5985=VERTEX_POINT ( 'NONE', #6795 ) ;
#6002=DIRECTION ( 'NONE',  ( -0.3505116388060184329, 0.000000000000000000, -0.9365583756827543516 ) ) ;
#6007=LINE ( 'NONE', #6108, #5401 ) ;
#6011=VERTEX_POINT ( 'NONE', #14756 ) ;
#6013=ORIENTED_EDGE ( 'NONE', *, *, #6841, .T. ) ;
#6016=LINE ( 'NONE', #7309, #4852 ) ;
#6020=LINE ( 'NONE', #7419, #4171 ) ;
#6022=FACE_BOUND ( 'NONE', #20993, .T. ) ;
#6029=DIRECTION ( 'NONE',  ( 0.000000000000000000, 0.000000000000000000, 1.000000000000000000 ) ) ;
#6035=EDGE_CURVE ( 'NONE', #5798, #10333, #6082, .T. ) ;
#6044=EDGE_CURVE ( 'NONE', #14946, #4339, #6917, .T. ) ;
#6050=EDGE_CURVE ( 'NONE', #14751, #15077, #11490, .T. ) ;
#6057=EDGE_CURVE ( 'NONE', #5712, #5798, #1136, .T. ) ;
#6058=ORIENTED_EDGE ( 'NONE', *, *, #17304, .T. ) ;
#6060=VERTEX_POINT ( 'NONE', #8018 ) ;
#6070=DIRECTION ( 'NONE',  ( -0.000000000000000000, -0.000000000000000000, -1.000000000000000000 ) ) ;
#6082=LINE ( 'NONE', #17871, #16268 ) ;
#6084=LINE ( 'NONE', #7493, #20518 ) ;
#6085=CIRCLE ( 'NONE', #14408, 21.20245194746113526 ) ;
#6088=FACE_OUTER_BOUND ( 'NONE', #20327, .T. ) ;
#6094=LINE ( 'NONE', #12499, #21382 ) ;
#6098=ADVANCED_FACE ( 'NONE', ( #14650 ), #9754, .F. ) ;
#6099=CIRCLE ( 'NONE', #956, 9.999999999999994671 ) ;
#6100=FACE_OUTER_BOUND ( 'NONE', #5610, .T. ) ;
#6105=CIRCLE ( 'NONE', #1286, 43.46661168214937732 ) ;
#6108=CARTESIAN_POINT ( 'NONE',  ( -49.57497958038185715, 160.1716627696692683, 50.00000000000000000 ) ) ;
#6119=DIRECTION ( 'NONE',  ( 1.232945044042657126E-32, -9.855701800883825964E-17, 1.000000000000000000 ) ) ;
#6123=DIRECTION ( 'NONE',  ( 0.000000000000000000, 0.000000000000000000, -1.000000000000000000 ) ) ;
#6126=CARTESIAN_POINT ( 'NONE',  ( -28.68588794268872633, 250.8848358243226357, 0.000000000000000000 ) ) ;
#6141=ORIENTED_EDGE ( 'NONE', *, *, #5457, .T. ) ;
#6142=ORIENTED_EDGE ( 'NONE', *, *, #13800, .T. ) ;
#6144=DIRECTION ( 'NONE',  ( 1.000000000000000000, 0.000000000000000000, 0.000000000000000000 ) ) ;
#6145=VERTEX_POINT ( 'NONE', #3283 ) ;
#6150=CARTESIAN_POINT ( 'NONE',  ( 71.32175588950862277, 75.31183677523708297, 94.99999999999994316 ) ) ;
#6157=CARTESIAN_POINT ( 'NONE',  ( 6.416697501590670427, 217.7548513357008630, 45.00000000000000000 ) ) ;
#6161=ORIENTED_EDGE ( 'NONE', *, *, #21293, .F. ) ;
#6175=VECTOR ( 'NONE', #2870, 1000.000000000000000 ) ;
#6183=CARTESIAN_POINT ( 'NONE',  ( -49.57497958038186425, 230.5765313837437418, -49.99999999999999289 ) ) ;
#6188=VECTOR ( 'NONE', #10482, 1000.000000000000000 ) ;
#6200=LINE ( 'NONE', #10961, #11368 ) ;
#6202=CARTESIAN_POINT ( 'NONE',  ( 6.416697501590670427, 172.9933428177121471, 45.00000000000000000 ) ) ;
#6204=PLANE ( 'NONE',  #20169 ) ;
#6205=CARTESIAN_POINT ( 'NONE',  ( 60.74769842942832554, 56.85652257517428865, 40.00000000000000000 ) ) ;
#6215=ORIENTED_EDGE ( 'NONE', *, *, #3113, .T. ) ;
#6218=ADVANCED_FACE ( 'NONE', ( #6727 ), #14864, .F. ) ;
#6225=CARTESIAN_POINT ( 'NONE',  ( -28.68588794268872633, 230.8848358243226073, 0.000000000000000000 ) ) ;
#6226=VECTOR ( 'NONE', #2436, 1000.000000000000000 ) ;
#6230=CARTESIAN_POINT ( 'NONE',  ( 51.50493485826542184, 170.1716627696692683, 20.00000000000000355 ) ) ;
#6234=PLANE ( 'NONE',  #7631 ) ;
#6238=FACE_OUTER_BOUND ( 'NONE', #504, .T. ) ;
#6239=CARTESIAN_POINT ( 'NONE',  ( -28.68588794268873698, 56.85652257517428865, 0.000000000000000000 ) ) ;
#6248=ORIENTED_EDGE ( 'NONE', *, *, #12533, .T. ) ;
#6250=CARTESIAN_POINT ( 'NONE',  ( 88.15330054274429017, 79.55187051032177692, 94.99999999999994316 ) ) ;
#6252=ORIENTED_EDGE ( 'NONE', *, *, #16463, .F. ) ;
#6265=FACE_OUTER_BOUND ( 'NONE', #7356, .T. ) ;
#6269=EDGE_LOOP ( 'NONE', ( #18718, #15425, #20276, #15241 ) ) ;
#6272=AXIS2_PLACEMENT_3D ( 'NONE', #20015, #7225, #16881 ) ;
#6282=DIRECTION ( 'NONE',  ( 0.000000000000000000, -1.000000000000000000, 0.000000000000000000 ) ) ;
#6289=VECTOR ( 'NONE', #14093, 1000.000000000000000 ) ;
#6295=CARTESIAN_POINT ( 'NONE',  ( 91.21585410611801592, 31.85652257517428865, -85.46735025547123143 ) ) ;
#6297=ORIENTED_EDGE ( 'NONE', *, *, #12814, .F. ) ;
#6298=CARTESIAN_POINT ( 'NONE',  ( -32.25189173780753293, 50.98147789719760681, 49.47307091579321536 ) ) ;
#6299=EDGE_CURVE ( 'NONE', #17635, #18850, #13875, .T. ) ;
#6313=DIRECTION ( 'NONE',  ( 0.000000000000000000, -0.000000000000000000, -1.000000000000000000 ) ) ;
#6318=AXIS2_PLACEMENT_3D ( 'NONE', #14048, #14375, #10884 ) ;
#6323=ORIENTED_EDGE ( 'NONE', *, *, #16235, .F. ) ;
#6328=AXIS2_PLACEMENT_3D ( 'NONE', #6351, #7546, #14171 ) ;
#6332=VECTOR ( 'NONE', #20828, 1000.000000000000000 ) ;
#6335=DIRECTION ( 'NONE',  ( 2.399110633850889130E-16, 0.000000000000000000, -1.000000000000000000 ) ) ;
#6342=CARTESIAN_POINT ( 'NONE',  ( 27.98965548446208373, 333.8848358243226357, 40.00000000000000000 ) ) ;
#6345=CARTESIAN_POINT ( 'NONE',  ( 65.85920792673738333, 160.1716627696692683, 20.00000000000000355 ) ) ;
#6351=CARTESIAN_POINT ( 'NONE',  ( 43.53705524234220547, -133.1434774248255906, -96.62835994548002816 ) ) ;
#6354=CARTESIAN_POINT ( 'NONE',  ( 51.98438129372387806, 56.85652257517428865, 117.7249735956185219 ) ) ;
#6356=VERTEX_POINT ( 'NONE', #15710 ) ;
#6370=EDGE_LOOP ( 'NONE', ( #1038, #426 ) ) ;
#6372=ORIENTED_EDGE ( 'NONE', *, *, #9426, .T. ) ;
#6391=CARTESIAN_POINT ( 'NONE',  ( 20.42502041961813930, 230.5765313837437418, -60.00000000000000000 ) ) ;
#6392=LINE ( 'NONE', #1543, #2997 ) ;
#6398=CARTESIAN_POINT ( 'NONE',  ( 60.03793209889851568, 30.52886280891152282, 131.1729372809869005 ) ) ;
#6404=DIRECTION ( 'NONE',  ( -0.000000000000000000, 1.000000000000000000, -0.000000000000000000 ) ) ;
#6409=CARTESIAN_POINT ( 'NONE',  ( -13.59795901728759482, 49.21534327078636295, 47.25690868943056699 ) ) ;
#6412=PLANE ( 'NONE',  #4579 ) ;
#6414=CARTESIAN_POINT ( 'NONE',  ( 115.7989814974898195, 160.1716627696691830, 20.00000000000000355 ) ) ;
#6420=CIRCLE ( 'NONE', #19915, 5.000000000000004441 ) ;
#6426=EDGE_CURVE ( 'NONE', #14255, #15845, #13529, .T. ) ;
#6427=ORIENTED_EDGE ( 'NONE', *, *, #20063, .F. ) ;
#6433=DIRECTION ( 'NONE',  ( -0.000000000000000000, -1.000000000000000000, -0.000000000000000000 ) ) ;
#6439=CARTESIAN_POINT ( 'NONE',  ( 125.7989814974898053, 10.52886280891152104, 40.00000000000000000 ) ) ;
#6440=DIRECTION ( 'NONE',  ( -1.000000000000000000, 0.000000000000000000, 0.000000000000000000 ) ) ;
#6441=CARTESIAN_POINT ( 'NONE',  ( 91.21585410611801592, 31.85652257517428865, 40.00000000000000000 ) ) ;
#6442=AXIS2_PLACEMENT_3D ( 'NONE', #14353, #6002, #17788 ) ;
#6463=VECTOR ( 'NONE', #6465, 1000.000000000000000 ) ;
#6465=DIRECTION ( 'NONE',  ( -0.000000000000000000, -0.000000000000000000, -1.000000000000000000 ) ) ;
#6468=CARTESIAN_POINT ( 'NONE',  ( 115.7989814974898337, 152.5259582928263740, -40.00000000000000000 ) ) ;
#6474=PLANE ( 'NONE',  #13626 ) ;
#6478=EDGE_LOOP ( 'NONE', ( #4210, #16583, #17593, #7571, #14863, #1612, #6372, #1211, #6801, #8122, #10737, #7522, #19925, #14309, #20623 ) ) ;
#6479=ORIENTED_EDGE ( 'NONE', *, *, #3225, .T. ) ;
#6490=LINE ( 'NONE', #4565, #19323 ) ;
#6495=CARTESIAN_POINT ( 'NONE',  ( 35.96497763894178945, 230.5765313837437418, 60.00000000000000000 ) ) ;
#6501=EDGE_CURVE ( 'NONE', #7438, #10209, #10129, .T. ) ;
#6506=DIRECTION ( 'NONE',  ( 0.000000000000000000, 0.000000000000000000, -1.000000000000000000 ) ) ;
#6507=ORIENTED_EDGE ( 'NONE', *, *, #6035, .T. ) ;
#6508=CARTESIAN_POINT ( 'NONE',  ( -32.89591654994843140, 52.24166481711759502, 49.42222731526657498 ) ) ;
#6509=AXIS2_PLACEMENT_3D ( 'NONE', #11041, #9428, #16046 ) ;
#6513=CARTESIAN_POINT ( 'NONE',  ( -28.68588794268872633, 174.3162933293988033, 0.000000000000000000 ) ) ;
#6519=FACE_OUTER_BOUND ( 'NONE', #20785, .T. ) ;
#6523=DIRECTION ( 'NONE',  ( -0.000000000000000000, 1.000000000000000000, -0.000000000000000000 ) ) ;
#6531=EDGE_LOOP ( 'NONE', ( #12619, #17533, #18014, #2397 ) ) ;
#6532=CARTESIAN_POINT ( 'NONE',  ( 81.24038404635966515, 30.52886280891152282, 94.99999999999994316 ) ) ;
#6542=DIRECTION ( 'NONE',  ( -1.000000000000000000, -0.000000000000000000, 0.000000000000000000 ) ) ;
#6543=VECTOR ( 'NONE', #3761, 1000.000000000000000 ) ;
#6549=PLANE ( 'NONE',  #9111 ) ;
#6550=CARTESIAN_POINT ( 'NONE',  ( 88.15330054274427596, 79.55187051032177692, -94.99999999999994316 ) ) ;
#6551=LINE ( 'NONE', #3431, #17644 ) ;
#6553=CARTESIAN_POINT ( 'NONE',  ( 2.416697501590669095, 217.7548513357008630, 45.00000000000000000 ) ) ;
#6566=CYLINDRICAL_SURFACE ( 'NONE', #6944, 21.20245194746113526 ) ;
#6567=ADVANCED_FACE ( 'NONE', ( #17089 ), #13634, .T. ) ;
#6571=VECTOR ( 'NONE', #18206, 1000.000000000000000 ) ;
#6572=CARTESIAN_POINT ( 'NONE',  ( 60.03793209889851568, 10.52886280891152104, 136.1729372809869005 ) ) ;
#6577=AXIS2_PLACEMENT_3D ( 'NONE', #20707, #14231, #5880 ) ;
#6578=VECTOR ( 'NONE', #19043, 1000.000000000000000 ) ;
#6582=CARTESIAN_POINT ( 'NONE',  ( -28.68588794268872633, 333.8848358243226357, 0.000000000000000000 ) ) ;
#6585=ORIENTED_EDGE ( 'NONE', *, *, #4721, .F. ) ;
#6586=ORIENTED_EDGE ( 'NONE', *, *, #17304, .F. ) ;
#6609=CIRCLE ( 'NONE', #2833, 22.72497359561857877 ) ;
#6616=CARTESIAN_POINT ( 'NONE',  ( -31.15442323855227968, 49.43082946763288277, 49.54048453831437371 ) ) ;
#6620=CYLINDRICAL_SURFACE ( 'NONE', #14218, 49.93977357075244328 ) ;
#6626=DIRECTION ( 'NONE',  ( -0.000000000000000000, -0.000000000000000000, -1.000000000000000000 ) ) ;
#6628=CARTESIAN_POINT ( 'NONE',  ( 81.24038404635966515, 30.52886280891152282, -94.99999999999994316 ) ) ;
#6646=EDGE_LOOP ( 'NONE', ( #19343, #6992, #7626, #706, #10661, #15345 ) ) ;
#6651=CARTESIAN_POINT ( 'NONE',  ( -11.50805310488956756, 52.75566815483727368, -46.53193503222628635 ) ) ;
#6656=PLANE ( 'NONE',  #19804 ) ;
#6657=CARTESIAN_POINT ( 'NONE',  ( 20.42502041961814641, 163.4113008177049835, -60.00000000000000000 ) ) ;
#6658=LINE ( 'NONE', #3002, #7037 ) ;
#6659=CIRCLE ( 'NONE', #11856, 10.00000000000000178 ) ;
#6661=CARTESIAN_POINT ( 'NONE',  ( -28.68588794268873698, 10.52886280891152104, 0.000000000000000000 ) ) ;
#6672=DIRECTION ( 'NONE',  ( 1.000000000000000000, 0.000000000000000000, 0.000000000000000000 ) ) ;
#6673=VERTEX_POINT ( 'NONE', #7220 ) ;
#6680=AXIS2_PLACEMENT_3D ( 'NONE', #3938, #7282, #2753 ) ;
#6690=LINE ( 'NONE', #11673, #8647 ) ;
#6698=ORIENTED_EDGE ( 'NONE', *, *, #18960, .F. ) ;
#6699=ORIENTED_EDGE ( 'NONE', *, *, #9663, .T. ) ;
#6701=DIRECTION ( 'NONE',  ( -0.000000000000000000, 0.000000000000000000, -1.000000000000000000 ) ) ;
#6702=AXIS2_PLACEMENT_3D ( 'NONE', #18407, #5109, #7143 ) ;
#6705=ORIENTED_EDGE ( 'NONE', *, *, #19806, .T. ) ;
#6710=ADVANCED_FACE ( 'NONE', ( #11005 ), #3015, .F. ) ;
#6718=PLANE ( 'NONE',  #12658 ) ;
#6727=FACE_OUTER_BOUND ( 'NONE', #6269, .T. ) ;
#6729=CARTESIAN_POINT ( 'NONE',  ( -32.69803402958404348, 51.81231153067828643, 49.43888967890881503 ) ) ;
#6738=CARTESIAN_POINT ( 'NONE',  ( -15.09323033528205116, 47.79017490167774440, 47.70849690890445771 ) ) ;
#6740=PLANE ( 'NONE',  #12906 ) ;
#6752=VERTEX_POINT ( 'NONE', #2915 ) ;
#6758=ORIENTED_EDGE ( 'NONE', *, *, #11205, .T. ) ;
#6761=EDGE_CURVE ( 'NONE', #15845, #17381, #1862, .T. ) ;
#6764=DIRECTION ( 'NONE',  ( -3.836511174089486173E-16, 0.000000000000000000, 1.000000000000000000 ) ) ;
#6765=DIRECTION ( 'NONE',  ( 0.000000000000000000, 0.000000000000000000, -1.000000000000000000 ) ) ;
#6767=DIRECTION ( 'NONE',  ( -0.000000000000000000, -0.000000000000000000, 1.000000000000000000 ) ) ;
#6770=CARTESIAN_POINT ( 'NONE',  ( 292.4526463419396691, 308.2087638784415162, 20.00000000000000355 ) ) ;
#6772=CARTESIAN_POINT ( 'NONE',  ( -33.70050622342144209, 54.95587029918029742, -49.34681548815472496 ) ) ;
#6779=ORIENTED_EDGE ( 'NONE', *, *, #17085, .T. ) ;
#6785=EDGE_CURVE ( 'NONE', #17432, #14968, #21073, .T. ) ;
#6786=AXIS2_PLACEMENT_3D ( 'NONE', #15464, #12207, #18794 ) ;
#6793=AXIS2_PLACEMENT_3D ( 'NONE', #16823, #11622, #9987 ) ;
#6794=CARTESIAN_POINT ( 'NONE',  ( 81.24038404635966515, 30.52886280891152282, -94.99999999999994316 ) ) ;
#6795=CARTESIAN_POINT ( 'NONE',  ( 115.7989814974898337, 152.5259582928263740, 20.00000000000000355 ) ) ;
#6801=ORIENTED_EDGE ( 'NONE', *, *, #11277, .F. ) ;
#6803=ORIENTED_EDGE ( 'NONE', *, *, #10400, .F. ) ;
#6807=ORIENTED_EDGE ( 'NONE', *, *, #9452, .F. ) ;
#6809=AXIS2_PLACEMENT_3D ( 'NONE', #2896, #19428, #12521 ) ;
#6813=VECTOR ( 'NONE', #13112, 1000.000000000000000 ) ;
#6815=CARTESIAN_POINT ( 'NONE',  ( 78.68120802659203150, 149.7457237375499517, -20.00000000000000355 ) ) ;
#6829=EDGE_LOOP ( 'NONE', ( #5736, #954, #5902, #16079, #10977 ) ) ;
#6841=EDGE_CURVE ( 'NONE', #10209, #5504, #4608, .T. ) ;
#6844=PLANE ( 'NONE',  #15819 ) ;
#6855=CIRCLE ( 'NONE', #18946, 5.000000000000004441 ) ;
#6856=ORIENTED_EDGE ( 'NONE', *, *, #113, .T. ) ;
#6858=ORIENTED_EDGE ( 'NONE', *, *, #12606, .T. ) ;
#6864=EDGE_LOOP ( 'NONE', ( #18490, #12003, #12514, #20568, #123, #7663, #10814, #6252 ) ) ;
#6866=CARTESIAN_POINT ( 'NONE',  ( -17.27797297620858430, 46.45732233689483337, -48.27343946592336010 ) ) ;
#6871=LINE ( 'NONE', #15333, #2518 ) ;
#6874=CARTESIAN_POINT ( 'NONE',  ( 78.68120802659203150, 149.7457237375499517, 20.00000000000000355 ) ) ;
#6879=CARTESIAN_POINT ( 'NONE',  ( -33.81853030400259996, 55.90295019273428068, -49.33467926027583417 ) ) ;
#6902=CIRCLE ( 'NONE', #19005, 40.00000000000000000 ) ;
#6908=EDGE_LOOP ( 'NONE', ( #15554, #20119, #13420, #15263 ) ) ;
#6911=CARTESIAN_POINT ( 'NONE',  ( 51.50493485826542184, 141.8799693780962912, 20.00000000000000355 ) ) ;
#6917=CIRCLE ( 'NONE', #16961, 5.000000000000004441 ) ;
#6922=CARTESIAN_POINT ( 'NONE',  ( -30.69714544437698933, 48.92315038370448121, 121.1724415244209894 ) ) ;
#6925=VECTOR ( 'NONE', #3316, 1000.000000000000000 ) ;
#6927=EDGE_CURVE ( 'NONE', #3730, #19453, #606, .T. ) ;
#6934=VECTOR ( 'NONE', #14245, 1000.000000000000000 ) ;
#6935=VECTOR ( 'NONE', #1905, 1000.000000000000000 ) ;
#6944=AXIS2_PLACEMENT_3D ( 'NONE', #13187, #18144, #14203 ) ;
#6949=CARTESIAN_POINT ( 'NONE',  ( -123.2946569474810161, 10.52886280891152104, 20.57735571454641388 ) ) ;
#6965=ORIENTED_EDGE ( 'NONE', *, *, #10809, .T. ) ;
#6972=CARTESIAN_POINT ( 'NONE',  ( 88.28695088269886071, 142.5259582928263455, 40.00000000000000000 ) ) ;
#6973=EDGE_CURVE ( 'NONE', #19853, #18701, #3831, .T. ) ;
#6978=PLANE ( 'NONE',  #9757 ) ;
#6980=EDGE_CURVE ( 'NONE', #4584, #8426, #19721, .T. ) ;
#6982=LINE ( 'NONE', #17160, #19035 ) ;
#6988=EDGE_CURVE ( 'NONE', #604, #7438, #7017, .T. ) ;
#6989=ORIENTED_EDGE ( 'NONE', *, *, #7093, .T. ) ;
#6992=ORIENTED_EDGE ( 'NONE', *, *, #440, .T. ) ;
#6998=CARTESIAN_POINT ( 'NONE',  ( 105.7989814974898479, 152.5259582928263740, -20.00000000000000355 ) ) ;
#7005=EDGE_CURVE ( 'NONE', #13483, #11839, #21325, .T. ) ;
#7008=CARTESIAN_POINT ( 'NONE',  ( -28.68588794268872633, 333.8848358243226357, 0.000000000000000000 ) ) ;
#7010=ORIENTED_EDGE ( 'NONE', *, *, #9347, .T. ) ;
#7017=CIRCLE ( 'NONE', #19127, 49.93977357075243617 ) ;
#7023=EDGE_CURVE ( 'NONE', #2702, #8292, #9781, .T. ) ;
#7025=CARTESIAN_POINT ( 'NONE',  ( 30.42502041961814996, 170.1716627696692683, -20.00000000000000355 ) ) ;
#7029=CARTESIAN_POINT ( 'NONE',  ( -26.36214243864212037, 46.04536198394939106, 122.1890418585359015 ) ) ;
#7034=ORIENTED_EDGE ( 'NONE', *, *, #8610, .F. ) ;
#7037=VECTOR ( 'NONE', #21061, 1000.000000000000114 ) ;
#7052=EDGE_CURVE ( 'NONE', #4231, #4363, #7377, .T. ) ;
#7061=DIRECTION ( 'NONE',  ( 1.000000000000000000, 0.000000000000000000, -0.000000000000000000 ) ) ;
#7064=EDGE_LOOP ( 'NONE', ( #8965, #19966 ) ) ;
#7066=ORIENTED_EDGE ( 'NONE', *, *, #11701, .F. ) ;
#7075=DIRECTION ( 'NONE',  ( -1.000000000000000000, 0.000000000000000000, 0.000000000000000000 ) ) ;
#7084=CARTESIAN_POINT ( 'NONE',  ( 105.7989814974898479, 152.5259582928263740, -20.00000000000000355 ) ) ;
#7089=EDGE_LOOP ( 'NONE', ( #3966, #18540, #895, #14020, #4094, #7886 ) ) ;
#7093=EDGE_CURVE ( 'NONE', #5985, #2702, #4044, .T. ) ;
#7097=DIRECTION ( 'NONE',  ( -0.1337298367054296222, 0.9910178256594273094, -0.000000000000000000 ) ) ;
#7099=ORIENTED_EDGE ( 'NONE', *, *, #11004, .F. ) ;
#7103=DIRECTION ( 'NONE',  ( 1.000000000000000000, 0.000000000000000000, 0.000000000000000000 ) ) ;
#7105=EDGE_CURVE ( 'NONE', #12056, #17482, #17146, .T. ) ;
#7118=ORIENTED_EDGE ( 'NONE', *, *, #8627, .T. ) ;
#7129=CARTESIAN_POINT ( 'NONE',  ( 60.03793209889851568, 30.52886280891152282, 126.1729372809868863 ) ) ;
#7141=EDGE_LOOP ( 'NONE', ( #13419, #5842, #14415 ) ) ;
#7142=ORIENTED_EDGE ( 'NONE', *, *, #13867, .T. ) ;
#7143=DIRECTION ( 'NONE',  ( 0.000000000000000000, -0.000000000000000000, 1.000000000000000000 ) ) ;
#7146=VECTOR ( 'NONE', #15813, 1000.000000000000000 ) ;
#7148=CARTESIAN_POINT ( 'NONE',  ( 52.60622592008805043, 10.52886280891152104, 151.0302712373927250 ) ) ;
#7149=ADVANCED_FACE ( 'NONE', ( #10850, #15637, #17454, #12271, #2642 ), #20495, .F. ) ;
#7161=DIRECTION ( 'NONE',  ( -0.000000000000000000, -1.000000000000000000, -0.000000000000000000 ) ) ;
#7163=CARTESIAN_POINT ( 'NONE',  ( -25.99280818006741356, 45.91387061696119076, -122.2681842339391523 ) ) ;
#7169=ORIENTED_EDGE ( 'NONE', *, *, #17728, .T. ) ;
#7179=DIRECTION ( 'NONE',  ( 0.000000000000000000, 0.9253149302858357794, 0.3791995250394160633 ) ) ;
#7183=ADVANCED_FACE ( 'NONE', ( #19188 ), #17562, .F. ) ;
#7188=AXIS2_PLACEMENT_3D ( 'NONE', #5914, #9154, #2900 ) ;
#7190=CARTESIAN_POINT ( 'NONE',  ( 60.03793209889851568, 30.52886280891152282, 136.1729372809869005 ) ) ;
#7194=EDGE_CURVE ( 'NONE', #5288, #12191, #6084, .T. ) ;
#7213=AXIS2_PLACEMENT_3D ( 'NONE', #10374, #5299, #15063 ) ;
#7215=EDGE_CURVE ( 'NONE', #18669, #15822, #10475, .T. ) ;
#7220=CARTESIAN_POINT ( 'NONE',  ( -22.30770786884144741, 45.31613216062291372, -122.9933582338429687 ) ) ;
#7222=EDGE_LOOP ( 'NONE', ( #2358, #15533, #17072, #317 ) ) ;
#7225=DIRECTION ( 'NONE',  ( 0.000000000000000000, 0.000000000000000000, 1.000000000000000000 ) ) ;
#7226=EDGE_LOOP ( 'NONE', ( #714, #5366, #6807, #2509 ) ) ;
#7237=CARTESIAN_POINT ( 'NONE',  ( -27.39625443478472278, 46.47175521496745176, 121.9628765649355415 ) ) ;
#7245=ORIENTED_EDGE ( 'NONE', *, *, #12879, .F. ) ;
#7267=LINE ( 'NONE', #2207, #3014 ) ;
#7269=CARTESIAN_POINT ( 'NONE',  ( 10.41669750159067220, 172.9933428177121471, 45.00000000000000000 ) ) ;
#7273=PLANE ( 'NONE',  #15448 ) ;
#7279=ORIENTED_EDGE ( 'NONE', *, *, #10583, .F. ) ;
#7282=DIRECTION ( 'NONE',  ( -0.000000000000000000, -0.000000000000000000, -1.000000000000000000 ) ) ;
#7290=DIRECTION ( 'NONE',  ( 0.000000000000000000, -0.000000000000000000, -1.000000000000000000 ) ) ;
#7305=VERTEX_POINT ( 'NONE', #9444 ) ;
#7309=CARTESIAN_POINT ( 'NONE',  ( 30.42502041961813575, 271.1055109169419097, -20.00000000000000355 ) ) ;
#7311=ORIENTED_EDGE ( 'NONE', *, *, #18119, .T. ) ;
#7312=CARTESIAN_POINT ( 'NONE',  ( -49.57497958038186425, 230.5765313837437418, -49.99999999999999289 ) ) ;
#7326=DIRECTION ( 'NONE',  ( 0.000000000000000000, 1.000000000000000000, 0.000000000000000000 ) ) ;
#7328=ORIENTED_EDGE ( 'NONE', *, *, #14580, .F. ) ;
#7342=LINE ( 'NONE', #3785, #5296 ) ;
#7343=EDGE_CURVE ( 'NONE', #11949, #14089, #10144, .T. ) ;
#7348=CARTESIAN_POINT ( 'NONE',  ( 60.03793209889851568, 10.52886280891152104, -131.1729372809869005 ) ) ;
#7356=EDGE_LOOP ( 'NONE', ( #11946, #18267, #7010, #7837 ) ) ;
#7361=AXIS2_PLACEMENT_3D ( 'NONE', #7925, #60, #14554 ) ;
#7363=EDGE_CURVE ( 'NONE', #11681, #15032, #8399, .T. ) ;
#7376=EDGE_CURVE ( 'NONE', #15497, #12829, #5163, .T. ) ;
#7377=CIRCLE ( 'NONE', #6680, 10.00000000000000178 ) ;
#7380=DIRECTION ( 'NONE',  ( -8.881784197001252323E-16, 0.000000000000000000, 1.000000000000000000 ) ) ;
#7381=AXIS2_PLACEMENT_3D ( 'NONE', #1708, #11214, #17812 ) ;
#7382=CARTESIAN_POINT ( 'NONE',  ( -33.77124986504215087, 55.31983858414345434, -120.3516843130412468 ) ) ;
#7387=ORIENTED_EDGE ( 'NONE', *, *, #19182, .T. ) ;
#7391=CARTESIAN_POINT ( 'NONE',  ( -162.2727221670389781, 30.52886280891152282, -4.999999999999990230 ) ) ;
#7395=DIRECTION ( 'NONE',  ( 1.000000000000000000, 0.000000000000000000, 0.000000000000000000 ) ) ;
#7396=VECTOR ( 'NONE', #19502, 1000.000000000000000 ) ;
#7398=CARTESIAN_POINT ( 'NONE',  ( 51.98438129372387806, -133.1434774248255906, 94.99999999999994316 ) ) ;
#7400=DIRECTION ( 'NONE',  ( 0.008660258604321402487, -0.3791853047755957551, -0.9252802302887190855 ) ) ;
#7401=DIRECTION ( 'NONE',  ( -0.000000000000000000, -0.000000000000000000, 1.000000000000000000 ) ) ;
#7414=EDGE_CURVE ( 'NONE', #15822, #18669, #8411, .T. ) ;
#7419=CARTESIAN_POINT ( 'NONE',  ( -28.68588794268874054, 271.1055109169419666, 40.00000000000000000 ) ) ;
#7422=PLANE ( 'NONE',  #9459 ) ;
#7429=LINE ( 'NONE', #1078, #10571 ) ;
#7433=CARTESIAN_POINT ( 'NONE',  ( -18.68588794268873698, 281.1055109169419666, 20.00000000000000355 ) ) ;
#7438=VERTEX_POINT ( 'NONE', #10131 ) ;
#7439=ORIENTED_EDGE ( 'NONE', *, *, #12040, .F. ) ;
#7441=LINE ( 'NONE', #14067, #20789 ) ;
#7457=ORIENTED_EDGE ( 'NONE', *, *, #11510, .T. ) ;
#7459=EDGE_LOOP ( 'NONE', ( #16832, #17796, #21363, #2724 ) ) ;
#7479=PLANE ( 'NONE',  #3153 ) ;
#7480=CARTESIAN_POINT ( 'NONE',  ( 163.6892970195449948, 191.6575133381268756, -49.76543245040357277 ) ) ;
#7488=CIRCLE ( 'NONE', #10248, 4.999999999999990230 ) ;
#7489=VERTEX_POINT ( 'NONE', #12400 ) ;
#7493=CARTESIAN_POINT ( 'NONE',  ( 164.2593879927715932, 166.6963511708817691, 60.00000000000000000 ) ) ;
#7496=DIRECTION ( 'NONE',  ( 9.855701800883827197E-17, -1.000000000000000000, 9.855701800883827197E-17 ) ) ;
#7497=CYLINDRICAL_SURFACE ( 'NONE', #6577, 40.00000000000000000 ) ;
#7501=CARTESIAN_POINT ( 'NONE',  ( 69.55160839065807465, 152.8169032537915086, 64.80145223029053625 ) ) ;
#7506=CARTESIAN_POINT ( 'NONE',  ( 163.6892970195449948, 191.6575133381268756, 49.76543245040357277 ) ) ;
#7508=VECTOR ( 'NONE', #1624, 1000.000000000000000 ) ;
#7522=ORIENTED_EDGE ( 'NONE', *, *, #10059, .F. ) ;
#7532=CARTESIAN_POINT ( 'NONE',  ( 78.68120802659203150, 149.7457237375499517, -66.14548919766382085 ) ) ;
#7545=ORIENTED_EDGE ( 'NONE', *, *, #15811, .T. ) ;
#7546=DIRECTION ( 'NONE',  ( -0.3717199501173604759, 0.000000000000000000, 0.9283449136418786551 ) ) ;
#7551=VERTEX_POINT ( 'NONE', #14144 ) ;
#7553=EDGE_LOOP ( 'NONE', ( #19047, #7782, #13593, #8296, #14811, #2484 ) ) ;
#7557=CARTESIAN_POINT ( 'NONE',  ( -28.68588794268872633, 250.8848358243226357, 40.00000000000000000 ) ) ;
#7560=AXIS2_PLACEMENT_3D ( 'NONE', #8916, #15537, #7290 ) ;
#7562=CARTESIAN_POINT ( 'NONE',  ( 116.0391604516428430, 192.9550247130592027, 40.00000000000000000 ) ) ;
#7569=DIRECTION ( 'NONE',  ( 9.855701800883827197E-17, -1.000000000000000000, 9.855701800883827197E-17 ) ) ;
#7571=ORIENTED_EDGE ( 'NONE', *, *, #17240, .T. ) ;
#7583=DIRECTION ( 'NONE',  ( -1.000000000000000000, 0.000000000000000000, 0.000000000000000000 ) ) ;
#7587=DIRECTION ( 'NONE',  ( 0.000000000000000000, -1.000000000000000000, 0.000000000000000000 ) ) ;
#7594=ORIENTED_EDGE ( 'NONE', *, *, #12639, .F. ) ;
#7602=ORIENTED_EDGE ( 'NONE', *, *, #12926, .F. ) ;
#7614=VECTOR ( 'NONE', #9639, 1000.000000000000114 ) ;
#7618=EDGE_CURVE ( 'NONE', #11300, #17480, #10647, .T. ) ;
#7623=AXIS2_PLACEMENT_3D ( 'NONE', #12522, #4298, #15880 ) ;
#7626=ORIENTED_EDGE ( 'NONE', *, *, #2898, .F. ) ;
#7631=AXIS2_PLACEMENT_3D ( 'NONE', #6342, #21171, #4723 ) ;
#7632=VECTOR ( 'NONE', #3925, 1000.000000000000000 ) ;
#7633=VERTEX_POINT ( 'NONE', #20942 ) ;
#7636=VERTEX_POINT ( 'NONE', #11402 ) ;
#7639=EDGE_CURVE ( 'NONE', #4929, #17485, #11196, .T. ) ;
#7643=FACE_BOUND ( 'NONE', #3906, .T. ) ;
#7644=ADVANCED_BREP_SHAPE_REPRESENTATION ( '', ( #11152, #12794 ), #32 ) ;
#7649=EDGE_CURVE ( 'NONE', #18462, #6752, #1340, .T. ) ;
#7654=CARTESIAN_POINT ( 'NONE',  ( -18.68588794268873698, 281.1055109169419666, 40.00000000000000000 ) ) ;
#7656=CARTESIAN_POINT ( 'NONE',  ( 29.72350413846044859, 280.4463447002762564, 40.00000000000000000 ) ) ;
#7658=VERTEX_POINT ( 'NONE', #17692 ) ;
#7661=ORIENTED_EDGE ( 'NONE', *, *, #17122, .T. ) ;
#7663=ORIENTED_EDGE ( 'NONE', *, *, #5129, .F. ) ;
#7665=VECTOR ( 'NONE', #17468, 1000.000000000000000 ) ;
#7673=DIRECTION ( 'NONE',  ( 0.000000000000000000, 0.000000000000000000, -1.000000000000000000 ) ) ;
#7674=CARTESIAN_POINT ( 'NONE',  ( 30.42502041961813575, 271.1055109169419097, 40.00000000000000000 ) ) ;
#7678=ORIENTED_EDGE ( 'NONE', *, *, #19607, .T. ) ;
#7707=ORIENTED_EDGE ( 'NONE', *, *, #607, .F. ) ;
#7709=ORIENTED_EDGE ( 'NONE', *, *, #17690, .F. ) ;
#7710=DIRECTION ( 'NONE',  ( -0.9997392892938121722, -0.02283316540262222971, 0.000000000000000000 ) ) ;
#7717=DIRECTION ( 'NONE',  ( 1.000000000000000000, 0.000000000000000000, 0.000000000000000000 ) ) ;
#7720=DIRECTION ( 'NONE',  ( 0.000000000000000000, 1.000000000000000000, 0.000000000000000000 ) ) ;
#7723=VECTOR ( 'NONE', #20420, 1000.000000000000000 ) ;
#7726=CARTESIAN_POINT ( 'NONE',  ( 30.42502041961814996, 180.1716627696692967, -20.00000000000000355 ) ) ;
#7732=ORIENTED_EDGE ( 'NONE', *, *, #19059, .T. ) ;
#7738=EDGE_LOOP ( 'NONE', ( #2114, #184, #15688, #13403, #7940, #15079, #18691, #18537, #19710, #549, #12942, #20649 ) ) ;
#7741=ORIENTED_EDGE ( 'NONE', *, *, #19490, .F. ) ;
#7743=LINE ( 'NONE', #21374, #8656 ) ;
#7752=ADVANCED_FACE ( 'NONE', ( #4604 ), #21364, .T. ) ;
#7755=EDGE_CURVE ( 'NONE', #13610, #12221, #7936, .T. ) ;
#7765=CARTESIAN_POINT ( 'NONE',  ( 6.416697501590670427, 217.7548513357008630, -45.00000000000000000 ) ) ;
#7778=DIRECTION ( 'NONE',  ( -0.000000000000000000, -0.000000000000000000, 1.000000000000000000 ) ) ;
#7779=EDGE_LOOP ( 'NONE', ( #12548, #17248, #20353 ) ) ;
#7782=ORIENTED_EDGE ( 'NONE', *, *, #16824, .T. ) ;
#7801=ADVANCED_FACE ( 'NONE', ( #14424 ), #13217, .T. ) ;
#7807=VERTEX_POINT ( 'NONE', #19584 ) ;
#7810=EDGE_CURVE ( 'NONE', #6752, #18462, #6855, .T. ) ;
#7812=CIRCLE ( 'NONE', #3670, 53.46661168214943416 ) ;
#7819=DIRECTION ( 'NONE',  ( 1.000000000000000000, 0.000000000000000000, 0.000000000000000000 ) ) ;
#7821=CARTESIAN_POINT ( 'NONE',  ( 81.24038404635965094, 30.52886280891152282, 131.1729372809869005 ) ) ;
#7826=CARTESIAN_POINT ( 'NONE',  ( 2.416697501590669095, 217.7548513357008630, -60.00000000000000000 ) ) ;
#7829=ADVANCED_FACE ( 'NONE', ( #12893 ), #11254, .T. ) ;
#7830=VECTOR ( 'NONE', #20482, 1000.000000000000114 ) ;
#7837=ORIENTED_EDGE ( 'NONE', *, *, #19528, .F. ) ;
#7841=DIRECTION ( 'NONE',  ( 0.000000000000000000, -1.000000000000000000, 0.000000000000000000 ) ) ;
#7843=ORIENTED_EDGE ( 'NONE', *, *, #7810, .F. ) ;
#7845=FACE_OUTER_BOUND ( 'NONE', #9778, .T. ) ;
#7858=DIRECTION ( 'NONE',  ( 1.000000000000000000, 0.000000000000000000, 0.000000000000000000 ) ) ;
#7864=VERTEX_POINT ( 'NONE', #9423 ) ;
#7866=PLANE ( 'NONE',  #14929 ) ;
#7879=AXIS2_PLACEMENT_3D ( 'NONE', #6532, #9570, #16509 ) ;
#7880=ADVANCED_FACE ( 'NONE', ( #15244 ), #8835, .F. ) ;
#7886=ORIENTED_EDGE ( 'NONE', *, *, #7005, .F. ) ;
#7894=DIRECTION ( 'NONE',  ( 0.000000000000000000, -1.000000000000000000, 0.000000000000000000 ) ) ;
#7901=CARTESIAN_POINT ( 'NONE',  ( -28.68588794268872633, 250.8848358243226357, 0.000000000000000000 ) ) ;
#7903=AXIS2_PLACEMENT_3D ( 'NONE', #6225, #12840, #19535 ) ;
#7909=ORIENTED_EDGE ( 'NONE', *, *, #12457, .T. ) ;
#7912=DIRECTION ( 'NONE',  ( 0.000000000000000000, -1.000000000000000000, 0.000000000000000000 ) ) ;
#7915=FACE_OUTER_BOUND ( 'NONE', #6864, .T. ) ;
#7921=DIRECTION ( 'NONE',  ( -0.000000000000000000, -0.000000000000000000, -1.000000000000000000 ) ) ;
#7923=DIRECTION ( 'NONE',  ( 0.000000000000000000, 0.000000000000000000, 1.000000000000000000 ) ) ;
#7925=CARTESIAN_POINT ( 'NONE',  ( -49.57497958038184294, -6.743947802724785386E-15, 0.000000000000000000 ) ) ;
#7933=AXIS2_PLACEMENT_3D ( 'NONE', #4150, #13689, #2328 ) ;
#7936=LINE ( 'NONE', #4921, #15848 ) ;
#7940=ORIENTED_EDGE ( 'NONE', *, *, #16463, .T. ) ;
#7949=DIRECTION ( 'NONE',  ( 0.000000000000000000, -1.000000000000000000, 0.000000000000000000 ) ) ;
#7952=AXIS2_PLACEMENT_3D ( 'NONE', #5005, #20041, #8127 ) ;
#7954=LINE ( 'NONE', #4720, #15008 ) ;
#7957=AXIS2_PLACEMENT_3D ( 'NONE', #19429, #11411, #6123 ) ;
#7962=EDGE_CURVE ( 'NONE', #14472, #16345, #8171, .T. ) ;
#7963=AXIS2_PLACEMENT_3D ( 'NONE', #6661, #8169, #8278 ) ;
#7971=DIRECTION ( 'NONE',  ( 0.000000000000000000, -0.000000000000000000, -1.000000000000000000 ) ) ;
#7973=AXIS2_PLACEMENT_3D ( 'NONE', #20312, #17073, #18468 ) ;
#7974=ORIENTED_EDGE ( 'NONE', *, *, #21080, .T. ) ;
#7981=LINE ( 'NONE', #14609, #20639 ) ;
#7988=CYLINDRICAL_SURFACE ( 'NONE', #10657, 18.29169339157296648 ) ;
#7991=ORIENTED_EDGE ( 'NONE', *, *, #1303, .F. ) ;
#8009=VECTOR ( 'NONE', #13211, 1000.000000000000000 ) ;
#8016=ADVANCED_FACE ( 'NONE', ( #857 ), #10240, .T. ) ;
#8018=CARTESIAN_POINT ( 'NONE',  ( 72.94945500224395118, 285.0140030772282103, 20.00000000000000355 ) ) ;
#8021=DIRECTION ( 'NONE',  ( -0.000000000000000000, -0.000000000000000000, -1.000000000000000000 ) ) ;
#8022=VECTOR ( 'NONE', #8165, 1000.000000000000000 ) ;
#8032=CARTESIAN_POINT ( 'NONE',  ( 115.7989814974898195, 160.1716627696691830, -20.00000000000000355 ) ) ;
#8036=CARTESIAN_POINT ( 'NONE',  ( 65.85920792673738333, 160.1716627696692683, 20.00000000000000355 ) ) ;
#8046=DIRECTION ( 'NONE',  ( -1.000000000000000000, 0.000000000000000000, 0.000000000000000000 ) ) ;
#8051=ORIENTED_EDGE ( 'NONE', *, *, #4123, .F. ) ;
#8055=ORIENTED_EDGE ( 'NONE', *, *, #13252, .F. ) ;
#8057=CYLINDRICAL_SURFACE ( 'NONE', #7957, 21.20245194746112105 ) ;
#8061=LINE ( 'NONE', #6439, #9772 ) ;
#8063=CARTESIAN_POINT ( 'NONE',  ( 20.42502041961814641, 160.1716627696692683, 60.00000000000000000 ) ) ;
#8069=CARTESIAN_POINT ( 'NONE',  ( -33.84809828339280102, 56.85652257517428865, -49.33155846391706945 ) ) ;
#8077=EDGE_CURVE ( 'NONE', #3125, #3575, #3741, .T. ) ;
#8085=CARTESIAN_POINT ( 'NONE',  ( -18.68588794268873698, 323.8848358243226357, 20.00000000000000355 ) ) ;
#8087=LINE ( 'NONE', #4966, #7508 ) ;
#8090=ADVANCED_FACE ( 'NONE', ( #6022, #10883 ), #20955, .F. ) ;
#8106=ADVANCED_FACE ( 'NONE', ( #2789 ), #19003, .T. ) ;
#8108=CARTESIAN_POINT ( 'NONE',  ( 27.98965548446208729, 333.8848358243226357, 40.00000000000000000 ) ) ;
#8110=PLANE ( 'NONE',  #1512 ) ;
#8112=CARTESIAN_POINT ( 'NONE',  ( -33.77147056149369320, 55.32675751745503590, 120.3516180215634819 ) ) ;
#8113=LINE ( 'NONE', #19917, #16628 ) ;
#8116=EDGE_CURVE ( 'NONE', #17381, #3413, #12411, .T. ) ;
#8119=ORIENTED_EDGE ( 'NONE', *, *, #15447, .T. ) ;
#8122=ORIENTED_EDGE ( 'NONE', *, *, #6050, .F. ) ;
#8125=PLANE ( 'NONE',  #3258 ) ;
#8127=DIRECTION ( 'NONE',  ( 0.000000000000000000, 0.000000000000000000, -1.000000000000000000 ) ) ;
#8128=FACE_OUTER_BOUND ( 'NONE', #2254, .T. ) ;
#8134=CARTESIAN_POINT ( 'NONE',  ( -17.74392196230863661, 46.24441999140541526, 48.38146745362002576 ) ) ;
#8142=VECTOR ( 'NONE', #1128, 1000.000000000000000 ) ;
#8147=EDGE_CURVE ( 'NONE', #9302, #1002, #12734, .T. ) ;
#8148=CIRCLE ( 'NONE', #9883, 220.7252770684331438 ) ;
#8149=EDGE_LOOP ( 'NONE', ( #6705, #7311, #11457, #7034 ) ) ;
#8154=VERTEX_POINT ( 'NONE', #4189 ) ;
#8157=EDGE_LOOP ( 'NONE', ( #12484, #13501, #3881, #2648, #1958, #17513, #1007, #11245, #3886, #6323 ) ) ;
#8163=DIRECTION ( 'NONE',  ( 1.000000000000000000, 0.000000000000000000, 0.000000000000000000 ) ) ;
#8165=DIRECTION ( 'NONE',  ( 0.000000000000000000, -1.000000000000000000, 0.000000000000000000 ) ) ;
#8167=VECTOR ( 'NONE', #9874, 1000.000000000000114 ) ;
#8169=DIRECTION ( 'NONE',  ( -0.000000000000000000, -1.000000000000000000, -0.000000000000000000 ) ) ;
#8171=( BOUNDED_CURVE ( )  B_SPLINE_CURVE ( 3, ( #17283, #4982, #20314, #2468 ),
 .UNSPECIFIED., .F., .T. ) 
 B_SPLINE_CURVE_WITH_KNOTS ( ( 4, 4 ),
 ( 3.164427803482926738, 4.712388980384689674 ),
 .UNSPECIFIED. ) 
 CURVE ( )  GEOMETRIC_REPRESENTATION_ITEM ( )  RATIONAL_B_SPLINE_CURVE ( ( 1.000000000000000000, 0.8100893075783975883, 0.8100893075783975883, 1.000000000000000000 ) ) 
 REPRESENTATION_ITEM ( '' )  );
#8181=EDGE_LOOP ( 'NONE', ( #3231, #871, #1526, #9066 ) ) ;
#8183=DIRECTION ( 'NONE',  ( 1.000000000000000000, 1.250996701150283068E-16, -0.000000000000000000 ) ) ;
#8185=ORIENTED_EDGE ( 'NONE', *, *, #7376, .F. ) ;
#8197=CARTESIAN_POINT ( 'NONE',  ( 6.416697501590670427, 217.7548513357008630, -49.99999999999999289 ) ) ;
#8200=ADVANCED_FACE ( 'NONE', ( #2574 ), #1270, .T. ) ;
#8201=CARTESIAN_POINT ( 'NONE',  ( -49.57497958038185715, 160.1716627696692683, 50.00000000000000000 ) ) ;
#8208=ORIENTED_EDGE ( 'NONE', *, *, #17543, .T. ) ;
#8224=AXIS2_PLACEMENT_3D ( 'NONE', #1323, #13104, #11359 ) ;
#8226=CARTESIAN_POINT ( 'NONE',  ( 107.6674317086782935, 187.4856410316723441, -20.00000000000000355 ) ) ;
#8246=CARTESIAN_POINT ( 'NONE',  ( -25.36425983038314058, 45.72515563955213480, 49.49023492600293395 ) ) ;
#8247=DIRECTION ( 'NONE',  ( 0.000000000000000000, -0.000000000000000000, 1.000000000000000000 ) ) ;
#8248=FACE_OUTER_BOUND ( 'NONE', #9939, .T. ) ;
#8249=DIRECTION ( 'NONE',  ( 1.000000000000000000, -0.000000000000000000, -0.000000000000000000 ) ) ;
#8256=CARTESIAN_POINT ( 'NONE',  ( 20.42502041961813930, 230.5765313837437418, 40.00000000000000000 ) ) ;
#8260=ORIENTED_EDGE ( 'NONE', *, *, #6761, .T. ) ;
#8264=CARTESIAN_POINT ( 'NONE',  ( 20.42502041961814641, 160.1716627696692683, -60.00000000000000000 ) ) ;
#8275=EDGE_CURVE ( 'NONE', #15561, #12697, #11639, .T. ) ;
#8278=DIRECTION ( 'NONE',  ( 0.000000000000000000, 0.000000000000000000, 1.000000000000000000 ) ) ;
#8280=DIRECTION ( 'NONE',  ( -0.000000000000000000, -0.000000000000000000, -1.000000000000000000 ) ) ;
#8285=VECTOR ( 'NONE', #13250, 1000.000000000000000 ) ;
#8287=EDGE_CURVE ( 'NONE', #15817, #18169, #14795, .T. ) ;
#8292=VERTEX_POINT ( 'NONE', #3528 ) ;
#8296=ORIENTED_EDGE ( 'NONE', *, *, #2966, .F. ) ;
#8297=DIRECTION ( 'NONE',  ( 0.000000000000000000, 0.000000000000000000, 1.000000000000000000 ) ) ;
#8302=AXIS2_PLACEMENT_3D ( 'NONE', #18102, #16712, #3298 ) ;
#8305=DIRECTION ( 'NONE',  ( 1.000000000000000000, 0.000000000000000000, 0.000000000000000000 ) ) ;
#8312=DIRECTION ( 'NONE',  ( 0.9365583756827543516, 0.000000000000000000, 0.3505116388060184329 ) ) ;
#8313=VERTEX_POINT ( 'NONE', #16629 ) ;
#8357=CARTESIAN_POINT ( 'NONE',  ( -162.2727221670389781, 10.52886280891152104, 0.000000000000000000 ) ) ;
#8360=CARTESIAN_POINT ( 'NONE',  ( 91.21585410611801592, 56.85652257517428865, -94.99999999999994316 ) ) ;
#8364=DIRECTION ( 'NONE',  ( 0.000000000000000000, 1.000000000000000000, 0.000000000000000000 ) ) ;
#8369=CIRCLE ( 'NONE', #14954, 20.00000000000000000 ) ;
#8372=EDGE_CURVE ( 'NONE', #2086, #1584, #653, .T. ) ;
#8378=ORIENTED_EDGE ( 'NONE', *, *, #14669, .T. ) ;
#8383=CARTESIAN_POINT ( 'NONE',  ( -11.91940135186754723, 51.80353952486193947, -46.68172999105591714 ) ) ;
#8387=DIRECTION ( 'NONE',  ( 0.000000000000000000, 0.000000000000000000, 1.000000000000000000 ) ) ;
#8388=DIRECTION ( 'NONE',  ( 0.000000000000000000, -0.000000000000000000, 1.000000000000000000 ) ) ;
#8396=CARTESIAN_POINT ( 'NONE',  ( -30.52044739588059841, 48.73524092274013242, -49.56800486934177741 ) ) ;
#8399=LINE ( 'NONE', #20197, #2907 ) ;
#8402=DIRECTION ( 'NONE',  ( 0.000000000000000000, 0.000000000000000000, 1.000000000000000000 ) ) ;
#8411=CIRCLE ( 'NONE', #1878, 4.000000000000003553 ) ;
#8417=VECTOR ( 'NONE', #3108, 1000.000000000000000 ) ;
#8425=ADVANCED_FACE ( 'NONE', ( #1925 ), #3634, .F. ) ;
#8426=VERTEX_POINT ( 'NONE', #8595 ) ;
#8428=ORIENTED_EDGE ( 'NONE', *, *, #717, .T. ) ;
#8439=DIRECTION ( 'NONE',  ( 0.000000000000000000, 0.000000000000000000, 1.000000000000000000 ) ) ;
#8446=DIRECTION ( 'NONE',  ( 0.000000000000000000, -1.000000000000000000, 0.000000000000000000 ) ) ;
#8454=ORIENTED_EDGE ( 'NONE', *, *, #9819, .F. ) ;
#8455=DIRECTION ( 'NONE',  ( 0.000000000000000000, 0.000000000000000000, 1.000000000000000000 ) ) ;
#8467=CARTESIAN_POINT ( 'NONE',  ( 40.42502041961814996, 180.1716627696692967, -20.00000000000000355 ) ) ;
#8471=EDGE_CURVE ( 'NONE', #1920, #16558, #15218, .T. ) ;
#8480=ORIENTED_EDGE ( 'NONE', *, *, #8950, .T. ) ;
#8482=ORIENTED_EDGE ( 'NONE', *, *, #17293, .F. ) ;
#8485=DIRECTION ( 'NONE',  ( -0.000000000000000000, -0.000000000000000000, -1.000000000000000000 ) ) ;
#8486=CARTESIAN_POINT ( 'NONE',  ( 43.53705524234220547, 30.52886280891152282, -96.62835994548002816 ) ) ;
#8490=CARTESIAN_POINT ( 'NONE',  ( -10.91048723079944871, 54.76430750887173105, -46.30741063304804328 ) ) ;
#8493=DIRECTION ( 'NONE',  ( 1.000000000000000000, 0.000000000000000000, 0.000000000000000000 ) ) ;
#8497=EDGE_CURVE ( 'NONE', #554, #739, #15864, .T. ) ;
#8502=CARTESIAN_POINT ( 'NONE',  ( 35.96497763894178945, 230.5765313837437418, 60.00000000000000000 ) ) ;
#8509=ORIENTED_EDGE ( 'NONE', *, *, #11412, .T. ) ;
#8517=EDGE_CURVE ( 'NONE', #15103, #554, #16840, .T. ) ;
#8523=AXIS2_PLACEMENT_3D ( 'NONE', #18243, #14912, #96 ) ;
#8525=CIRCLE ( 'NONE', #14426, 21.20245194746113526 ) ;
#8528=ORIENTED_EDGE ( 'NONE', *, *, #15056, .F. ) ;
#8530=ORIENTED_EDGE ( 'NONE', *, *, #8497, .T. ) ;
#8532=ORIENTED_EDGE ( 'NONE', *, *, #2046, .T. ) ;
#8537=EDGE_LOOP ( 'NONE', ( #16449, #20949, #10047, #16349 ) ) ;
#8539=VECTOR ( 'NONE', #12174, 1000.000000000000000 ) ;
#8542=AXIS2_PLACEMENT_3D ( 'NONE', #8197, #14933, #4 ) ;
#8550=DIRECTION ( 'NONE',  ( 0.000000000000000000, -0.000000000000000000, -1.000000000000000000 ) ) ;
#8556=ORIENTED_EDGE ( 'NONE', *, *, #2692, .F. ) ;
#8571=CARTESIAN_POINT ( 'NONE',  ( 60.03793209889851568, 30.52886280891152282, -131.1729372809869005 ) ) ;
#8586=ORIENTED_EDGE ( 'NONE', *, *, #1622, .F. ) ;
#8595=CARTESIAN_POINT ( 'NONE',  ( -162.2727221670389781, 30.52886280891152282, 20.57735571454641033 ) ) ;
#8596=FACE_OUTER_BOUND ( 'NONE', #2227, .T. ) ;
#8598=DIRECTION ( 'NONE',  ( -0.000000000000000000, -0.000000000000000000, -1.000000000000000000 ) ) ;
#8599=VECTOR ( 'NONE', #5459, 1000.000000000000000 ) ;
#8604=CARTESIAN_POINT ( 'NONE',  ( -22.30770786884144741, 45.31613216062291372, -122.9933582338429687 ) ) ;
#8610=EDGE_CURVE ( 'NONE', #5497, #2086, #2126, .T. ) ;
#8611=ORIENTED_EDGE ( 'NONE', *, *, #1234, .T. ) ;
#8613=DIRECTION ( 'NONE',  ( -0.000000000000000000, 1.000000000000000000, -0.000000000000000000 ) ) ;
#8627=EDGE_CURVE ( 'NONE', #20033, #9674, #615, .T. ) ;
#8628=CARTESIAN_POINT ( 'NONE',  ( 2.416697501590669095, 172.9933428177121471, 60.00000000000000000 ) ) ;
#8633=ADVANCED_FACE ( 'NONE', ( #10641, #2336 ), #13802, .F. ) ;
#8637=EDGE_LOOP ( 'NONE', ( #11329, #5847, #793, #14062 ) ) ;
#8645=VECTOR ( 'NONE', #15955, 1000.000000000000000 ) ;
#8647=VECTOR ( 'NONE', #18264, 1000.000000000000000 ) ;
#8653=CARTESIAN_POINT ( 'NONE',  ( 35.96497763894178945, 230.5765313837437418, 40.00000000000000000 ) ) ;
#8656=VECTOR ( 'NONE', #6542, 1000.000000000000000 ) ;
#8657=DIRECTION ( 'NONE',  ( 1.000000000000000000, 0.000000000000000000, 0.000000000000000000 ) ) ;
#8667=CARTESIAN_POINT ( 'NONE',  ( 51.50493485826542184, 170.1716627696692683, -57.52045949366692668 ) ) ;
#8684=DIRECTION ( 'NONE',  ( -0.9283449136418786551, 0.000000000000000000, 0.3717199501173604759 ) ) ;
#8686=FACE_OUTER_BOUND ( 'NONE', #3829, .T. ) ;
#8688=EDGE_CURVE ( 'NONE', #16558, #13685, #6094, .T. ) ;
#8693=EDGE_LOOP ( 'NONE', ( #14513, #18376, #20125, #19899 ) ) ;
#8695=ORIENTED_EDGE ( 'NONE', *, *, #19490, .T. ) ;
#8698=ADVANCED_FACE ( 'NONE', ( #4486 ), #2546, .F. ) ;
#8699=VERTEX_POINT ( 'NONE', #7821 ) ;
#8704=CARTESIAN_POINT ( 'NONE',  ( -12.69441680977503850, 50.46651949346903621, -46.95261769007076680 ) ) ;
#8710=LINE ( 'NONE', #14907, #1129 ) ;
#8712=VECTOR ( 'NONE', #1594, 1000.000000000000000 ) ;
#8714=LINE ( 'NONE', #9907, #13367 ) ;
#8716=CARTESIAN_POINT ( 'NONE',  ( -162.2727221670389781, 30.52886280891152282, 4.999999999999990230 ) ) ;
#8717=VECTOR ( 'NONE', #4083, 1000.000000000000000 ) ;
#8719=EDGE_LOOP ( 'NONE', ( #7707, #18963, #3651, #18993 ) ) ;
#8720=DIRECTION ( 'NONE',  ( 0.000000000000000000, -1.000000000000000000, 0.000000000000000000 ) ) ;
#8727=ORIENTED_EDGE ( 'NONE', *, *, #4215, .F. ) ;
#8731=DIRECTION ( 'NONE',  ( 1.000000000000000000, 0.000000000000000000, 0.000000000000000000 ) ) ;
#8750=ORIENTED_EDGE ( 'NONE', *, *, #11205, .F. ) ;
#8758=VECTOR ( 'NONE', #13249, 1000.000000000000000 ) ;
#8761=LINE ( 'NONE', #15381, #6188 ) ;
#8765=EDGE_CURVE ( 'NONE', #16030, #15737, #15961, .T. ) ;
#8771=ORIENTED_EDGE ( 'NONE', *, *, #3353, .F. ) ;
#8777=CARTESIAN_POINT ( 'NONE',  ( -28.68588794268872633, 333.8848358243226357, 20.00000000000000000 ) ) ;
#8793=DIRECTION ( 'NONE',  ( -1.000000000000000000, -0.000000000000000000, 0.000000000000000000 ) ) ;
#8794=CARTESIAN_POINT ( 'NONE',  ( 2.416697501590669095, 217.7548513357008630, -45.00000000000000000 ) ) ;
#8795=CARTESIAN_POINT ( 'NONE',  ( 60.69669829156632090, 56.85652257517428865, 94.99999999999994316 ) ) ;
#8797=DIRECTION ( 'NONE',  ( -0.000000000000000000, -0.000000000000000000, -1.000000000000000000 ) ) ;
#8800=ORIENTED_EDGE ( 'NONE', *, *, #14210, .F. ) ;
#8804=CARTESIAN_POINT ( 'NONE',  ( 118.4271928232701043, 10.52886280891152104, 40.00000000000000000 ) ) ;
#8806=LINE ( 'NONE', #19082, #16255 ) ;
#8813=CARTESIAN_POINT ( 'NONE',  ( 60.03793209889851568, 30.52886280891152282, -126.1729372809868863 ) ) ;
#8823=PLANE ( 'NONE',  #11289 ) ;
#8825=ORIENTED_EDGE ( 'NONE', *, *, #20644, .T. ) ;
#8831=ORIENTED_EDGE ( 'NONE', *, *, #1836, .T. ) ;
#8832=CARTESIAN_POINT ( 'NONE',  ( 30.42502041961814285, 230.5765313837437418, -40.00000000000000000 ) ) ;
#8835=CYLINDRICAL_SURFACE ( 'NONE', #323, 9.999999999999994671 ) ;
#8845=DIRECTION ( 'NONE',  ( 1.000000000000000000, 0.000000000000000000, -0.000000000000000000 ) ) ;
#8855=ORIENTED_EDGE ( 'NONE', *, *, #5982, .F. ) ;
#8876=CIRCLE ( 'NONE', #973, 20.00000000000000000 ) ;
#8877=VERTEX_POINT ( 'NONE', #8032 ) ;
#8879=ORIENTED_EDGE ( 'NONE', *, *, #13966, .F. ) ;
#8880=DIRECTION ( 'NONE',  ( 1.000000000000000000, 1.250996701150283068E-16, -0.000000000000000000 ) ) ;
#8893=FACE_OUTER_BOUND ( 'NONE', #17387, .T. ) ;
#8898=EDGE_CURVE ( 'NONE', #2506, #16623, #16389, .T. ) ;
#8900=CARTESIAN_POINT ( 'NONE',  ( -26.35054759312642503, 46.04092669597897469, -122.1915506529835653 ) ) ;
#8903=VERTEX_POINT ( 'NONE', #13134 ) ;
#8909=CARTESIAN_POINT ( 'NONE',  ( 292.4526463419396691, 308.2087638784415162, -20.00000000000000355 ) ) ;
#8916=CARTESIAN_POINT ( 'NONE',  ( -162.2727221670389781, 30.52886280891152282, 0.000000000000000000 ) ) ;
#8920=CARTESIAN_POINT ( 'NONE',  ( 10.41669750159067220, 172.9933428177121471, -60.00000000000000000 ) ) ;
#8922=DIRECTION ( 'NONE',  ( -1.232945044042657126E-32, 9.855701800883825964E-17, 1.000000000000000000 ) ) ;
#8929=EDGE_LOOP ( 'NONE', ( #8482, #15368, #3698, #4039, #20463, #989 ) ) ;
#8931=ORIENTED_EDGE ( 'NONE', *, *, #3638, .T. ) ;
#8943=CARTESIAN_POINT ( 'NONE',  ( 115.7989814974898195, 160.1716627696691830, 20.00000000000000355 ) ) ;
#8948=EDGE_CURVE ( 'NONE', #16161, #258, #15629, .T. ) ;
#8950=EDGE_CURVE ( 'NONE', #16730, #8313, #12046, .T. ) ;
#8952=EDGE_CURVE ( 'NONE', #19571, #6011, #4107, .T. ) ;
#8956=EDGE_LOOP ( 'NONE', ( #8985, #14170, #18827, #12435 ) ) ;
#8961=CYLINDRICAL_SURFACE ( 'NONE', #17327, 4.000000000000001776 ) ;
#8963=EDGE_CURVE ( 'NONE', #4099, #4363, #13354, .T. ) ;
#8965=ORIENTED_EDGE ( 'NONE', *, *, #21038, .F. ) ;
#8969=CARTESIAN_POINT ( 'NONE',  ( -18.68588794268873698, 323.8848358243226357, 40.00000000000000000 ) ) ;
#8979=ORIENTED_EDGE ( 'NONE', *, *, #2184, .T. ) ;
#8985=ORIENTED_EDGE ( 'NONE', *, *, #11593, .F. ) ;
#8986=ORIENTED_EDGE ( 'NONE', *, *, #2295, .F. ) ;
#8987=DIRECTION ( 'NONE',  ( 1.000000000000000000, 0.000000000000000000, 0.000000000000000000 ) ) ;
#8998=CARTESIAN_POINT ( 'NONE',  ( 65.85920792673738333, 160.1716627696692683, -20.00000000000000355 ) ) ;
#9002=CARTESIAN_POINT ( 'NONE',  ( 118.4271928232701043, 10.52886280891152104, -40.00000000000000000 ) ) ;
#9003=DIRECTION ( 'NONE',  ( 1.374938938973709817E-16, -1.000000000000000000, 0.000000000000000000 ) ) ;
#9021=EDGE_CURVE ( 'NONE', #15047, #2858, #5540, .T. ) ;
#9023=DIRECTION ( 'NONE',  ( -0.000000000000000000, -0.000000000000000000, 1.000000000000000000 ) ) ;
#9032=CARTESIAN_POINT ( 'NONE',  ( -28.68588794268872277, 333.8848358243226357, -20.00000000000000000 ) ) ;
#9035=LINE ( 'NONE', #17377, #17502 ) ;
#9042=EDGE_LOOP ( 'NONE', ( #6058, #16133, #12293, #20673 ) ) ;
#9045=ORIENTED_EDGE ( 'NONE', *, *, #4427, .F. ) ;
#9046=LINE ( 'NONE', #12301, #1767 ) ;
#9056=VECTOR ( 'NONE', #1214, 1000.000000000000000 ) ;
#9064=ORIENTED_EDGE ( 'NONE', *, *, #12639, .T. ) ;
#9066=ORIENTED_EDGE ( 'NONE', *, *, #19266, .F. ) ;
#9069=LINE ( 'NONE', #17512, #14572 ) ;
#9070=ORIENTED_EDGE ( 'NONE', *, *, #17868, .F. ) ;
#9072=ORIENTED_EDGE ( 'NONE', *, *, #17082, .T. ) ;
#9079=DIRECTION ( 'NONE',  ( -0.000000000000000000, -0.000000000000000000, 1.000000000000000000 ) ) ;
#9084=CARTESIAN_POINT ( 'NONE',  ( -162.2727221670389781, 30.52886280891152282, 0.000000000000000000 ) ) ;
#9085=ADVANCED_FACE ( 'NONE', ( #8893 ), #15302, .F. ) ;
#9093=ORIENTED_EDGE ( 'NONE', *, *, #5521, .T. ) ;
#9111=AXIS2_PLACEMENT_3D ( 'NONE', #4824, #11421, #19329 ) ;
#9116=ORIENTED_EDGE ( 'NONE', *, *, #18810, .F. ) ;
#9121=CARTESIAN_POINT ( 'NONE',  ( 20.42502041961813930, 230.5765313837437418, 49.99999999999999289 ) ) ;
#9124=ORIENTED_EDGE ( 'NONE', *, *, #12814, .T. ) ;
#9129=CARTESIAN_POINT ( 'NONE',  ( 125.7989814974898337, 160.1716627696691830, 40.00000000000000000 ) ) ;
#9132=DIRECTION ( 'NONE',  ( 0.9997392892938120612, 0.02283316540262222277, -0.000000000000000000 ) ) ;
#9134=EDGE_CURVE ( 'NONE', #7636, #16109, #15090, .T. ) ;
#9138=CYLINDRICAL_SURFACE ( 'NONE', #4367, 4.999999999999990230 ) ;
#9142=VERTEX_POINT ( 'NONE', #11929 ) ;
#9144=ORIENTED_EDGE ( 'NONE', *, *, #18949, .T. ) ;
#9149=EDGE_LOOP ( 'NONE', ( #1941, #12407, #527, #3774 ) ) ;
#9152=EDGE_CURVE ( 'NONE', #15607, #8903, #13888, .T. ) ;
#9154=DIRECTION ( 'NONE',  ( -0.000000000000000000, -0.000000000000000000, -1.000000000000000000 ) ) ;
#9162=DIRECTION ( 'NONE',  ( 0.000000000000000000, -1.000000000000000000, 0.000000000000000000 ) ) ;
#9164=ADVANCED_FACE ( 'NONE', ( #3607 ), #2003, .F. ) ;
#9170=ORIENTED_EDGE ( 'NONE', *, *, #11264, .T. ) ;
#9171=ORIENTED_EDGE ( 'NONE', *, *, #1780, .T. ) ;
#9186=VECTOR ( 'NONE', #17552, 1000.000000000000000 ) ;
#9187=DIRECTION ( 'NONE',  ( -1.000000000000000000, 0.000000000000000000, 0.000000000000000000 ) ) ;
#9194=ORIENTED_EDGE ( 'NONE', *, *, #20063, .T. ) ;
#9196=ORIENTED_EDGE ( 'NONE', *, *, #18597, .T. ) ;
#9200=AXIS2_PLACEMENT_3D ( 'NONE', #6345, #14277, #7858 ) ;
#9205=ADVANCED_FACE ( 'NONE', ( #3708 ), #9317, .T. ) ;
#9208=EDGE_CURVE ( 'NONE', #8877, #13368, #10663, .T. ) ;
#9209=VECTOR ( 'NONE', #5785, 1000.000000000000000 ) ;
#9211=DIRECTION ( 'NONE',  ( 0.000000000000000000, 0.000000000000000000, 1.000000000000000000 ) ) ;
#9216=FACE_OUTER_BOUND ( 'NONE', #9916, .T. ) ;
#9224=AXIS2_PLACEMENT_3D ( 'NONE', #20560, #10810, #2392 ) ;
#9228=ORIENTED_EDGE ( 'NONE', *, *, #2966, .T. ) ;
#9231=DIRECTION ( 'NONE',  ( -1.000000000000000000, 0.000000000000000000, 0.000000000000000000 ) ) ;
#9245=CARTESIAN_POINT ( 'NONE',  ( -49.57497958038186425, 230.5765313837437418, 49.99999999999999289 ) ) ;
#9246=CARTESIAN_POINT ( 'NONE',  ( -28.68588794268872988, 47.23886018424757083, -49.60091809715359545 ) ) ;
#9251=DIRECTION ( 'NONE',  ( -0.000000000000000000, -0.000000000000000000, -1.000000000000000000 ) ) ;
#9254=ORIENTED_EDGE ( 'NONE', *, *, #219, .T. ) ;
#9259=ADVANCED_FACE ( 'NONE', ( #15725 ), #10721, .F. ) ;
#9263=PLANE ( 'NONE',  #7623 ) ;
#9267=CARTESIAN_POINT ( 'NONE',  ( 0.000000000000000000, 0.000000000000000000, 60.00000000000000000 ) ) ;
#9276=EDGE_CURVE ( 'NONE', #1881, #17507, #10618, .T. ) ;
#9285=CARTESIAN_POINT ( 'NONE',  ( -74.06037022053952512, 10.52886280891152104, 40.00000000000000000 ) ) ;
#9290=EDGE_CURVE ( 'NONE', #13610, #19679, #3767, .T. ) ;
#9294=APPLICATION_CONTEXT ( 'automotive_design' ) ;
#9296=CARTESIAN_POINT ( 'NONE',  ( 30.42502041961814996, 180.1716627696692967, -40.00000000000000000 ) ) ;
#9298=CYLINDRICAL_SURFACE ( 'NONE', #10451, 4.999999999999990230 ) ;
#9302=VERTEX_POINT ( 'NONE', #12682 ) ;
#9310=CARTESIAN_POINT ( 'NONE',  ( 2.416697501590669095, 217.7548513357008630, 49.99999999999999289 ) ) ;
#9317=CYLINDRICAL_SURFACE ( 'NONE', #671, 53.46661168214943416 ) ;
#9331=DIRECTION ( 'NONE',  ( 0.000000000000000000, 1.000000000000000000, 0.000000000000000000 ) ) ;
#9333=DIRECTION ( 'NONE',  ( -1.250996701150283068E-16, 1.000000000000000000, 0.000000000000000000 ) ) ;
#9336=ORIENTED_EDGE ( 'NONE', *, *, #17938, .T. ) ;
#9341=VECTOR ( 'NONE', #2006, 1000.000000000000000 ) ;
#9345=CARTESIAN_POINT ( 'NONE',  ( -162.2727221670389781, 10.52886280891152104, 4.999999999999990230 ) ) ;
#9347=EDGE_CURVE ( 'NONE', #12450, #12520, #18617, .T. ) ;
#9349=AXIS2_PLACEMENT_3D ( 'NONE', #11764, #16964, #3653 ) ;
#9359=VECTOR ( 'NONE', #20529, 1000.000000000000000 ) ;
#9370=ORIENTED_EDGE ( 'NONE', *, *, #16824, .F. ) ;
#9372=VERTEX_POINT ( 'NONE', #23 ) ;
#9385=VECTOR ( 'NONE', #17094, 1000.000000000000000 ) ;
#9390=EDGE_LOOP ( 'NONE', ( #11197, #16654, #17322, #11352 ) ) ;
#9392=VERTEX_POINT ( 'NONE', #8108 ) ;
#9394=CARTESIAN_POINT ( 'NONE',  ( 107.6674317086782935, 187.4856410316723441, -40.00000000000000000 ) ) ;
#9401=DIRECTION ( 'NONE',  ( -1.000000000000000000, 0.000000000000000000, 0.000000000000000000 ) ) ;
#9411=LINE ( 'NONE', #1413, #12227 ) ;
#9418=DIRECTION ( 'NONE',  ( 0.000000000000000000, 0.000000000000000000, 1.000000000000000000 ) ) ;
#9423=CARTESIAN_POINT ( 'NONE',  ( 81.24038404635965094, 30.52886280891152282, -131.1729372809869005 ) ) ;
#9426=EDGE_CURVE ( 'NONE', #19050, #12773, #20408, .T. ) ;
#9428=DIRECTION ( 'NONE',  ( 0.000000000000000000, 0.000000000000000000, 1.000000000000000000 ) ) ;
#9431=CARTESIAN_POINT ( 'NONE',  ( 91.21585410611801592, 31.85652257517428865, 40.00000000000000000 ) ) ;
#9444=CARTESIAN_POINT ( 'NONE',  ( -49.57497958038186425, 230.5765313837437418, -60.00000000000000000 ) ) ;
#9452=EDGE_CURVE ( 'NONE', #2936, #12320, #21221, .T. ) ;
#9459=AXIS2_PLACEMENT_3D ( 'NONE', #9267, #20632, #12199 ) ;
#9468=DIRECTION ( 'NONE',  ( 0.000000000000000000, -1.000000000000000000, 0.000000000000000000 ) ) ;
#9474=FACE_OUTER_BOUND ( 'NONE', #9886, .T. ) ;
#9476=ORIENTED_EDGE ( 'NONE', *, *, #717, .F. ) ;
#9478=DIRECTION ( 'NONE',  ( 1.776356839400250465E-15, 0.000000000000000000, 1.000000000000000000 ) ) ;
#9481=DIRECTION ( 'NONE',  ( 1.000000000000000000, 0.000000000000000000, 0.000000000000000000 ) ) ;
#9485=EDGE_CURVE ( 'NONE', #10233, #16560, #6490, .T. ) ;
#9498=CARTESIAN_POINT ( 'NONE',  ( -22.30770786884145451, 56.85652257517428865, -152.3753892284480003 ) ) ;
#9514=ORIENTED_EDGE ( 'NONE', *, *, #20422, .T. ) ;
#9533=LINE ( 'NONE', #10942, #9186 ) ;
#9538=EDGE_CURVE ( 'NONE', #18164, #10102, #11473, .T. ) ;
#9539=VECTOR ( 'NONE', #9003, 1000.000000000000000 ) ;
#9540=ORIENTED_EDGE ( 'NONE', *, *, #11811, .F. ) ;
#9541=CARTESIAN_POINT ( 'NONE',  ( 60.03793209889851568, 30.52886280891152282, -131.1729372809869005 ) ) ;
#9542=ORIENTED_EDGE ( 'NONE', *, *, #7052, .F. ) ;
#9552=FACE_OUTER_BOUND ( 'NONE', #8181, .T. ) ;
#9554=CARTESIAN_POINT ( 'NONE',  ( -11.05500197003667751, 54.24389605313263019, 46.36189423322173297 ) ) ;
#9559=CIRCLE ( 'NONE', #20269, 49.60091809715359545 ) ;
#9560=DIRECTION ( 'NONE',  ( 0.000000000000000000, 0.000000000000000000, -1.000000000000000000 ) ) ;
#9563=VECTOR ( 'NONE', #16546, 1000.000000000000000 ) ;
#9568=EDGE_CURVE ( 'NONE', #12017, #5497, #9841, .T. ) ;
#9569=EDGE_LOOP ( 'NONE', ( #14836, #17561, #8979, #19111 ) ) ;
#9570=DIRECTION ( 'NONE',  ( 1.000000000000000000, 0.000000000000000000, 3.836511174089486666E-16 ) ) ;
#9575=VERTEX_POINT ( 'NONE', #9634 ) ;
#9580=CARTESIAN_POINT ( 'NONE',  ( 91.21585410611801592, 56.85652257517428865, 85.46735025547120301 ) ) ;
#9587=PLANE ( 'NONE',  #1487 ) ;
#9592=DIRECTION ( 'NONE',  ( -0.000000000000000000, 1.000000000000000000, -0.000000000000000000 ) ) ;
#9593=DIRECTION ( 'NONE',  ( -0.000000000000000000, -0.000000000000000000, 1.000000000000000000 ) ) ;
#9609=CARTESIAN_POINT ( 'NONE',  ( 118.4271928232701043, 31.85652257517428865, 40.00000000000000000 ) ) ;
#9613=EDGE_CURVE ( 'NONE', #7633, #5562, #12765, .T. ) ;
#9622=ORIENTED_EDGE ( 'NONE', *, *, #10107, .T. ) ;
#9634=CARTESIAN_POINT ( 'NONE',  ( -33.84809828339280102, 56.85652257517428865, 49.33155846391706945 ) ) ;
#9639=DIRECTION ( 'NONE',  ( 1.157565925312684532E-16, -0.9253149302858357794, -0.3791995250394160633 ) ) ;
#9640=AXIS2_PLACEMENT_3D ( 'NONE', #5564, #17048, #7395 ) ;
#9647=ORIENTED_EDGE ( 'NONE', *, *, #14730, .F. ) ;
#9650=DIRECTION ( 'NONE',  ( 0.000000000000000000, 0.000000000000000000, -1.000000000000000000 ) ) ;
#9653=CARTESIAN_POINT ( 'NONE',  ( -22.30770786884145451, 30.52886280891152282, -122.9933582338429972 ) ) ;
#9663=EDGE_CURVE ( 'NONE', #739, #20672, #1049, .T. ) ;
#9672=ORIENTED_EDGE ( 'NONE', *, *, #3210, .F. ) ;
#9673=CARTESIAN_POINT ( 'NONE',  ( 60.03793209889851568, 10.52886280891152104, -131.1729372809869005 ) ) ;
#9674=VERTEX_POINT ( 'NONE', #10058 ) ;
#9683=CARTESIAN_POINT ( 'NONE',  ( 51.50493485826542184, 170.1716627696692683, 20.00000000000000355 ) ) ;
#9692=CARTESIAN_POINT ( 'NONE',  ( 6.416697501590670427, 217.7548513357008630, -45.00000000000000000 ) ) ;
#9693=ADVANCED_FACE ( 'NONE', ( #16887 ), #18390, .T. ) ;
#9706=ORIENTED_EDGE ( 'NONE', *, *, #1523, .T. ) ;
#9709=AXIS2_PLACEMENT_3D ( 'NONE', #2147, #2677, #1171 ) ;
#9717=LINE ( 'NONE', #8085, #18900 ) ;
#9720=CARTESIAN_POINT ( 'NONE',  ( 20.42502041961813575, 262.6374945681020563, 19.33651958906945012 ) ) ;
#9722=DIRECTION ( 'NONE',  ( 0.000000000000000000, -0.000000000000000000, 1.000000000000000000 ) ) ;
#9723=VERTEX_POINT ( 'NONE', #3579 ) ;
#9725=ORIENTED_EDGE ( 'NONE', *, *, #9613, .F. ) ;
#9726=ORIENTED_EDGE ( 'NONE', *, *, #5783, .T. ) ;
#9728=DIRECTION ( 'NONE',  ( 0.000000000000000000, 0.000000000000000000, -1.000000000000000000 ) ) ;
#9742=EDGE_CURVE ( 'NONE', #1881, #11167, #16681, .T. ) ;
#9753=VERTEX_POINT ( 'NONE', #10168 ) ;
#9754=CYLINDRICAL_SURFACE ( 'NONE', #13162, 5.000000000000004441 ) ;
#9755=ORIENTED_EDGE ( 'NONE', *, *, #16425, .F. ) ;
#9756=CARTESIAN_POINT ( 'NONE',  ( -33.38506921610404277, 53.58597874041705467, 49.37795238679517951 ) ) ;
#9757=AXIS2_PLACEMENT_3D ( 'NONE', #5462, #11956, #18127 ) ;
#9762=CARTESIAN_POINT ( 'NONE',  ( 81.24038404635966515, 30.52886280891152282, -94.99999999999994316 ) ) ;
#9764=CARTESIAN_POINT ( 'NONE',  ( -20.71087849649029522, 45.41521113178804114, 48.95842151343376969 ) ) ;
#9766=DIRECTION ( 'NONE',  ( 1.000000000000000000, 0.000000000000000000, 0.000000000000000000 ) ) ;
#9772=VECTOR ( 'NONE', #18020, 1000.000000000000000 ) ;
#9778=EDGE_LOOP ( 'NONE', ( #21234, #3254, #105, #14258 ) ) ;
#9781=CIRCLE ( 'NONE', #493, 49.93977357075243617 ) ;
#9791=ADVANCED_FACE ( 'NONE', ( #5092 ), #16786, .F. ) ;
#9800=FACE_OUTER_BOUND ( 'NONE', #8693, .T. ) ;
#9807=VERTEX_POINT ( 'NONE', #6815 ) ;
#9815=DIRECTION ( 'NONE',  ( 0.000000000000000000, -1.000000000000000000, 0.000000000000000000 ) ) ;
#9819=EDGE_CURVE ( 'NONE', #5108, #10498, #3473, .T. ) ;
#9820=DIRECTION ( 'NONE',  ( -0.9910178256594274204, -0.1337298367054296500, 0.000000000000000000 ) ) ;
#9828=ORIENTED_EDGE ( 'NONE', *, *, #19394, .T. ) ;
#9831=ORIENTED_EDGE ( 'NONE', *, *, #8952, .F. ) ;
#9841=LINE ( 'NONE', #1648, #20357 ) ;
#9843=DIRECTION ( 'NONE',  ( 0.000000000000000000, 1.000000000000000000, 0.000000000000000000 ) ) ;
#9845=CARTESIAN_POINT ( 'NONE',  ( -33.22918226429612076, 53.10839921601173330, 120.5024273052909081 ) ) ;
#9846=CARTESIAN_POINT ( 'NONE',  ( 69.79185940953689737, 142.2976266388001250, 40.00000000000000000 ) ) ;
#9857=CYLINDRICAL_SURFACE ( 'NONE', #2230, 21.20245194746112105 ) ;
#9858=EDGE_CURVE ( 'NONE', #17432, #454, #8761, .T. ) ;
#9865=SHAPE_DEFINITION_REPRESENTATION ( #3032, #21199 ) ;
#9866=DIRECTION ( 'NONE',  ( 1.000000000000000000, 0.000000000000000000, 0.000000000000000000 ) ) ;
#9869=FACE_OUTER_BOUND ( 'NONE', #18229, .T. ) ;
#9874=DIRECTION ( 'NONE',  ( -0.4989387216749512355, -0.8666372666885295839, -0.000000000000000000 ) ) ;
#9883=AXIS2_PLACEMENT_3D ( 'NONE', #6770, #8280, #3325 ) ;
#9886=EDGE_LOOP ( 'NONE', ( #8986, #8586, #3590, #16348 ) ) ;
#9895=PLANE ( 'NONE',  #17983 ) ;
#9907=CARTESIAN_POINT ( 'NONE',  ( 35.96497763894178945, 230.5765313837437418, 60.00000000000000000 ) ) ;
#9914=AXIS2_PLACEMENT_3D ( 'NONE', #9930, #9820, #19355 ) ;
#9916=EDGE_LOOP ( 'NONE', ( #7974, #7118, #4806, #10076, #12551, #8727, #19420, #3621, #13271, #13618 ) ) ;
#9920=EDGE_LOOP ( 'NONE', ( #2895, #7602, #9, #13824 ) ) ;
#9930=CARTESIAN_POINT ( 'NONE',  ( 78.68120802659203150, 149.7457237375499517, 94.99999999999994316 ) ) ;
#9932=CARTESIAN_POINT ( 'NONE',  ( -22.30770786884145451, 30.52886280891152282, -122.9933582338429972 ) ) ;
#9937=VERTEX_POINT ( 'NONE', #7557 ) ;
#9939=EDGE_LOOP ( 'NONE', ( #9064, #21181, #10575, #2037 ) ) ;
#9943=LINE ( 'NONE', #4870, #11091 ) ;
#9955=AXIS2_PLACEMENT_3D ( 'NONE', #6126, #16199, #14155 ) ;
#9956=EDGE_CURVE ( 'NONE', #5552, #7489, #14183, .T. ) ;
#9970=CARTESIAN_POINT ( 'NONE',  ( -32.00363043698316545, 50.57999860063866038, 49.49059492257082127 ) ) ;
#9971=VECTOR ( 'NONE', #10405, 1000.000000000000000 ) ;
#9980=CARTESIAN_POINT ( 'NONE',  ( -12.15981775011844768, 51.33689851414709437, 46.76771730510184710 ) ) ;
#9984=FACE_OUTER_BOUND ( 'NONE', #16084, .T. ) ;
#9987=DIRECTION ( 'NONE',  ( 0.000000000000000000, 0.000000000000000000, 1.000000000000000000 ) ) ;
#9990=ORIENTED_EDGE ( 'NONE', *, *, #16431, .T. ) ;
#9992=ORIENTED_EDGE ( 'NONE', *, *, #15044, .F. ) ;
#9996=ORIENTED_EDGE ( 'NONE', *, *, #20302, .F. ) ;
#10002=CARTESIAN_POINT ( 'NONE',  ( -18.70454317747300976, 45.89000029780063272, -48.58690594643588412 ) ) ;
#10009=CARTESIAN_POINT ( 'NONE',  ( -33.84809828339279392, 55.89938081350750565, 49.33155846391708366 ) ) ;
#10035=CARTESIAN_POINT ( 'NONE',  ( 29.72350413846044859, 280.4463447002762564, 20.00000000000000355 ) ) ;
#10039=AXIS2_PLACEMENT_3D ( 'NONE', #840, #8922, #10645 ) ;
#10040=VECTOR ( 'NONE', #16050, 1000.000000000000000 ) ;
#10043=ORIENTED_EDGE ( 'NONE', *, *, #17756, .F. ) ;
#10046=CARTESIAN_POINT ( 'NONE',  ( 292.4526463419396691, 308.2087638784415162, 40.00000000000000000 ) ) ;
#10047=ORIENTED_EDGE ( 'NONE', *, *, #4843, .T. ) ;
#10048=EDGE_LOOP ( 'NONE', ( #10307, #12885, #610, #11634 ) ) ;
#10051=DIRECTION ( 'NONE',  ( -0.000000000000000000, -0.000000000000000000, -1.000000000000000000 ) ) ;
#10058=CARTESIAN_POINT ( 'NONE',  ( 35.96497763894179656, 170.1716627696692683, -57.37501161332323107 ) ) ;
#10059=EDGE_CURVE ( 'NONE', #17320, #12803, #17831, .T. ) ;
#10063=CARTESIAN_POINT ( 'NONE',  ( -28.05669753933457145, 46.82147536802074939, 121.8123201430361888 ) ) ;
#10066=CARTESIAN_POINT ( 'NONE',  ( 2.416697501590669095, 172.9933428177121471, -60.00000000000000000 ) ) ;
#10070=ORIENTED_EDGE ( 'NONE', *, *, #4843, .F. ) ;
#10071=AXIS2_PLACEMENT_3D ( 'NONE', #13169, #18129, #16743 ) ;
#10076=ORIENTED_EDGE ( 'NONE', *, *, #3454, .T. ) ;
#10086=DIRECTION ( 'NONE',  ( 0.000000000000000000, 0.000000000000000000, 1.000000000000000000 ) ) ;
#10088=DIRECTION ( 'NONE',  ( -0.000000000000000000, -0.000000000000000000, 1.000000000000000000 ) ) ;
#10093=CARTESIAN_POINT ( 'NONE',  ( 30.07572094023280940, 170.1716627696692683, 57.31989048965873934 ) ) ;
#10096=EDGE_CURVE ( 'NONE', #5934, #18961, #16927, .T. ) ;
#10102=VERTEX_POINT ( 'NONE', #6572 ) ;
#10104=VERTEX_POINT ( 'NONE', #4540 ) ;
#10107=EDGE_CURVE ( 'NONE', #10687, #2936, #11125, .T. ) ;
#10108=ORIENTED_EDGE ( 'NONE', *, *, #14790, .T. ) ;
#10111=AXIS2_PLACEMENT_3D ( 'NONE', #16491, #2001, #20049 ) ;
#10112=ORIENTED_EDGE ( 'NONE', *, *, #6299, .F. ) ;
#10114=CARTESIAN_POINT ( 'NONE',  ( -10.76731745429009734, 55.79702461148883685, -46.25122601329427852 ) ) ;
#10118=LINE ( 'NONE', #16740, #4948 ) ;
#10122=FACE_OUTER_BOUND ( 'NONE', #18059, .T. ) ;
#10129=CIRCLE ( 'NONE', #10461, 220.7252770684331438 ) ;
#10131=CARTESIAN_POINT ( 'NONE',  ( 107.6674317086782935, 187.4856410316723441, 40.00000000000000000 ) ) ;
#10138=ADVANCED_FACE ( 'NONE', ( #16019 ), #14399, .F. ) ;
#10144=CIRCLE ( 'NONE', #4959, 4.999999999999990230 ) ;
#10153=DIRECTION ( 'NONE',  ( 0.000000000000000000, 1.000000000000000000, 0.000000000000000000 ) ) ;
#10168=CARTESIAN_POINT ( 'NONE',  ( 81.24038404635966515, 10.52886280891152104, 94.99999999999994316 ) ) ;
#10181=CARTESIAN_POINT ( 'NONE',  ( 64.58676821086662301, 170.1716627696692683, -57.64290030256307062 ) ) ;
#10197=DIRECTION ( 'NONE',  ( -1.854788578061058554E-16, -1.000000000000000000, 0.000000000000000000 ) ) ;
#10209=VERTEX_POINT ( 'NONE', #14714 ) ;
#10212=ORIENTED_EDGE ( 'NONE', *, *, #4215, .T. ) ;
#10214=CARTESIAN_POINT ( 'NONE',  ( -12.99034458037978546, 50.04225476994710675, -47.05236843673905867 ) ) ;
#10224=EDGE_CURVE ( 'NONE', #19655, #20672, #5063, .T. ) ;
#10230=VERTEX_POINT ( 'NONE', #15247 ) ;
#10233=VERTEX_POINT ( 'NONE', #5275 ) ;
#10235=CARTESIAN_POINT ( 'NONE',  ( 10.41669750159067220, 172.9933428177121471, 60.00000000000000000 ) ) ;
#10238=PLANE ( 'NONE',  #7973 ) ;
#10240=CYLINDRICAL_SURFACE ( 'NONE', #1017, 10.00000000000000533 ) ;
#10242=CARTESIAN_POINT ( 'NONE',  ( -10.76731745429010090, 56.85652257517428865, -46.25122601329427141 ) ) ;
#10248=AXIS2_PLACEMENT_3D ( 'NONE', #20906, #7587, #14215 ) ;
#10256=ORIENTED_EDGE ( 'NONE', *, *, #12606, .F. ) ;
#10263=ORIENTED_EDGE ( 'NONE', *, *, #15717, .T. ) ;
#10307=ORIENTED_EDGE ( 'NONE', *, *, #7093, .F. ) ;
#10312=VERTEX_POINT ( 'NONE', #10242 ) ;
#10321=DIRECTION ( 'NONE',  ( 0.000000000000000000, 0.000000000000000000, -1.000000000000000000 ) ) ;
#10324=VECTOR ( 'NONE', #3502, 1000.000000000000000 ) ;
#10325=CARTESIAN_POINT ( 'NONE',  ( 6.416697501590670427, 217.7548513357008630, 45.00000000000000000 ) ) ;
#10326=EDGE_CURVE ( 'NONE', #17590, #11997, #17609, .T. ) ;
#10331=CARTESIAN_POINT ( 'NONE',  ( -33.84809828339280102, 56.85652257517428865, -49.33155846391706945 ) ) ;
#10333=VERTEX_POINT ( 'NONE', #18366 ) ;
#10342=VERTEX_POINT ( 'NONE', #15420 ) ;
#10343=CARTESIAN_POINT ( 'NONE',  ( 115.7989814974898195, 160.1716627696691830, -40.00000000000000000 ) ) ;
#10349=DIRECTION ( 'NONE',  ( 0.000000000000000000, 0.000000000000000000, 1.000000000000000000 ) ) ;
#10354=EDGE_CURVE ( 'NONE', #18169, #4442, #2222, .T. ) ;
#10361=VERTEX_POINT ( 'NONE', #8804 ) ;
#10373=AXIS2_PLACEMENT_3D ( 'NONE', #359, #11367, #19593 ) ;
#10374=CARTESIAN_POINT ( 'NONE',  ( 20.42502041961813575, 271.1055109169419666, 40.00000000000000000 ) ) ;
#10379=FACE_OUTER_BOUND ( 'NONE', #5882, .T. ) ;
#10386=ORIENTED_EDGE ( 'NONE', *, *, #12935, .F. ) ;
#10391=ORIENTED_EDGE ( 'NONE', *, *, #1982, .F. ) ;
#10392=DIRECTION ( 'NONE',  ( -0.000000000000000000, -0.000000000000000000, -1.000000000000000000 ) ) ;
#10400=EDGE_CURVE ( 'NONE', #17320, #1920, #18965, .T. ) ;
#10405=DIRECTION ( 'NONE',  ( -1.000000000000000000, 0.000000000000000000, -8.901024030850960568E-17 ) ) ;
#10412=DIRECTION ( 'NONE',  ( 0.000000000000000000, 0.000000000000000000, 1.000000000000000000 ) ) ;
#10417=ORIENTED_EDGE ( 'NONE', *, *, #19479, .T. ) ;
#10429=DIRECTION ( 'NONE',  ( -0.000000000000000000, 1.000000000000000000, -0.000000000000000000 ) ) ;
#10435=DIRECTION ( 'NONE',  ( 1.000000000000000000, 1.374938938973709817E-16, -0.000000000000000000 ) ) ;
#10446=EDGE_CURVE ( 'NONE', #5712, #15685, #4556, .T. ) ;
#10449=DIRECTION ( 'NONE',  ( 0.9283449136418786551, -0.000000000000000000, 0.3717199501173604204 ) ) ;
#10451=AXIS2_PLACEMENT_3D ( 'NONE', #9084, #12563, #5729 ) ;
#10458=LINE ( 'NONE', #20746, #8717 ) ;
#10461=AXIS2_PLACEMENT_3D ( 'NONE', #10046, #12319, #5818 ) ;
#10465=DIRECTION ( 'NONE',  ( 1.000000000000000000, 0.000000000000000000, 0.000000000000000000 ) ) ;
#10473=LINE ( 'NONE', #13639, #9385 ) ;
#10474=ORIENTED_EDGE ( 'NONE', *, *, #18466, .F. ) ;
#10475=CIRCLE ( 'NONE', #4623, 4.000000000000003553 ) ;
#10482=DIRECTION ( 'NONE',  ( 1.000000000000000000, 0.000000000000000000, -8.901024030850963034E-17 ) ) ;
#10485=CARTESIAN_POINT ( 'NONE',  ( -30.95117587177153951, 49.20052347319550989, 121.1077492336972909 ) ) ;
#10498=VERTEX_POINT ( 'NONE', #14628 ) ;
#10522=ORIENTED_EDGE ( 'NONE', *, *, #1836, .F. ) ;
#10524=CARTESIAN_POINT ( 'NONE',  ( 81.24038404635966515, -343.0245277843623057, -94.99999999999994316 ) ) ;
#10528=ORIENTED_EDGE ( 'NONE', *, *, #2692, .T. ) ;
#10534=CARTESIAN_POINT ( 'NONE',  ( 35.96497763894178945, 170.1716627696692683, -40.00000000000000000 ) ) ;
#10537=EDGE_CURVE ( 'NONE', #17482, #1165, #9943, .T. ) ;
#10538=ADVANCED_FACE ( 'NONE', ( #3043 ), #12889, .T. ) ;
#10541=CARTESIAN_POINT ( 'NONE',  ( -123.2946569474810161, 30.52886280891152282, 20.57735571454641388 ) ) ;
#10550=ORIENTED_EDGE ( 'NONE', *, *, #13867, .F. ) ;
#10571=VECTOR ( 'NONE', #14055, 1000.000000000000000 ) ;
#10575=ORIENTED_EDGE ( 'NONE', *, *, #6299, .T. ) ;
#10583=EDGE_CURVE ( 'NONE', #7305, #4929, #21212, .T. ) ;
#10584=AXIS2_PLACEMENT_3D ( 'NONE', #12291, #525, #5472 ) ;
#10608=VECTOR ( 'NONE', #20883, 1000.000000000000114 ) ;
#10610=LINE ( 'NONE', #5426, #13509 ) ;
#10618=LINE ( 'NONE', #2417, #3430 ) ;
#10633=DIRECTION ( 'NONE',  ( -0.000000000000000000, -1.000000000000000000, -0.000000000000000000 ) ) ;
#10634=CARTESIAN_POINT ( 'NONE',  ( -28.68588794268872633, 271.1055109169419666, 0.000000000000000000 ) ) ;
#10637=EDGE_LOOP ( 'NONE', ( #16883, #9755, #4475, #3385 ) ) ;
#10641=FACE_OUTER_BOUND ( 'NONE', #17360, .T. ) ;
#10642=LINE ( 'NONE', #17155, #19247 ) ;
#10645=DIRECTION ( 'NONE',  ( 0.000000000000000000, -1.000000000000000000, 0.000000000000000000 ) ) ;
#10647=CIRCLE ( 'NONE', #20685, 4.000000000000001776 ) ;
#10656=ADVANCED_FACE ( 'NONE', ( #11576 ), #18167, .F. ) ;
#10657=AXIS2_PLACEMENT_3D ( 'NONE', #1310, #16027, #16448 ) ;
#10661=ORIENTED_EDGE ( 'NONE', *, *, #1971, .F. ) ;
#10662=FACE_OUTER_BOUND ( 'NONE', #15140, .T. ) ;
#10663=CIRCLE ( 'NONE', #15184, 49.93977357075243617 ) ;
#10684=DIRECTION ( 'NONE',  ( 0.000000000000000000, 0.000000000000000000, 1.000000000000000000 ) ) ;
#10687=VERTEX_POINT ( 'NONE', #12987 ) ;
#10699=FACE_OUTER_BOUND ( 'NONE', #6908, .T. ) ;
#10703=ORIENTED_EDGE ( 'NONE', *, *, #5647, .F. ) ;
#10706=ORIENTED_EDGE ( 'NONE', *, *, #12926, .T. ) ;
#10707=LINE ( 'NONE', #4237, #9056 ) ;
#10721=CYLINDRICAL_SURFACE ( 'NONE', #13106, 20.00000000000000000 ) ;
#10723=( LENGTH_UNIT ( ) NAMED_UNIT ( * ) SI_UNIT ( .MILLI., .METRE. ) );
#10724=VECTOR ( 'NONE', #4614, 1000.000000000000000 ) ;
#10729=DIRECTION ( 'NONE',  ( -0.000000000000000000, -0.000000000000000000, -1.000000000000000000 ) ) ;
#10730=VECTOR ( 'NONE', #20188, 1000.000000000000000 ) ;
#10733=CARTESIAN_POINT ( 'NONE',  ( 81.24038404635966515, 30.52886280891152282, -94.99999999999994316 ) ) ;
#10737=ORIENTED_EDGE ( 'NONE', *, *, #219, .F. ) ;
#10745=EDGE_LOOP ( 'NONE', ( #20094, #13965 ) ) ;
#10764=ORIENTED_EDGE ( 'NONE', *, *, #10939, .F. ) ;
#10776=DIRECTION ( 'NONE',  ( 0.000000000000000000, 0.000000000000000000, -1.000000000000000000 ) ) ;
#10782=AXIS2_PLACEMENT_3D ( 'NONE', #14727, #19683, #4868 ) ;
#10788=CIRCLE ( 'NONE', #16684, 20.57735571454641033 ) ;
#10803=EDGE_CURVE ( 'NONE', #15800, #9575, #10473, .T. ) ;
#10809=EDGE_CURVE ( 'NONE', #15103, #17195, #19407, .T. ) ;
#10810=DIRECTION ( 'NONE',  ( 0.000000000000000000, 1.000000000000000000, -0.000000000000000000 ) ) ;
#10812=CARTESIAN_POINT ( 'NONE',  ( 2.416697501590669095, 172.9933428177121471, 50.00000000000000000 ) ) ;
#10814=ORIENTED_EDGE ( 'NONE', *, *, #3669, .F. ) ;
#10816=EDGE_CURVE ( 'NONE', #1524, #4442, #1442, .T. ) ;
#10818=EDGE_LOOP ( 'NONE', ( #16132, #12214, #9990, #3771, #6758, #5713, #2932 ) ) ;
#10821=EDGE_LOOP ( 'NONE', ( #17924, #14307, #12277, #9072 ) ) ;
#10824=AXIS2_PLACEMENT_3D ( 'NONE', #4908, #11504, #13356 ) ;
#10834=CARTESIAN_POINT ( 'NONE',  ( 88.28695088269886071, 152.5259582928263740, -40.00000000000000000 ) ) ;
#10839=LINE ( 'NONE', #4355, #7614 ) ;
#10850=FACE_BOUND ( 'NONE', #11814, .T. ) ;
#10861=DIRECTION ( 'NONE',  ( 0.000000000000000000, -1.000000000000000000, 0.000000000000000000 ) ) ;
#10865=LINE ( 'NONE', #14354, #6934 ) ;
#10867=LINE ( 'NONE', #12183, #5387 ) ;
#10869=CARTESIAN_POINT ( 'NONE',  ( 60.03793209889851568, 30.52886280891152282, 131.1729372809869005 ) ) ;
#10871=VERTEX_POINT ( 'NONE', #9394 ) ;
#10883=FACE_OUTER_BOUND ( 'NONE', #3597, .T. ) ;
#10884=DIRECTION ( 'NONE',  ( 1.000000000000000000, 0.000000000000000000, 0.000000000000000000 ) ) ;
#10885=FACE_BOUND ( 'NONE', #11735, .T. ) ;
#10887=EDGE_CURVE ( 'NONE', #10230, #14472, #9069, .T. ) ;
#10898=DIRECTION ( 'NONE',  ( 0.000000000000000000, 0.000000000000000000, 1.000000000000000000 ) ) ;
#10916=VECTOR ( 'NONE', #9592, 1000.000000000000000 ) ;
#10918=EDGE_LOOP ( 'NONE', ( #6013, #15229, #18613, #20284 ) ) ;
#10924=DIRECTION ( 'NONE',  ( 0.000000000000000000, -1.000000000000000000, 0.000000000000000000 ) ) ;
#10926=EDGE_CURVE ( 'NONE', #19050, #7551, #7441, .T. ) ;
#10929=CARTESIAN_POINT ( 'NONE',  ( 35.96497763894178945, 230.5765313837437418, -60.00000000000000000 ) ) ;
#10939=EDGE_CURVE ( 'NONE', #10361, #2882, #12755, .T. ) ;
#10940=CARTESIAN_POINT ( 'NONE',  ( 105.7989814974898479, 142.5259582928263455, 20.00000000000000355 ) ) ;
#10942=CARTESIAN_POINT ( 'NONE',  ( 10.41669750159067220, 172.9933428177121471, -45.00000000000000000 ) ) ;
#10943=AXIS2_PLACEMENT_3D ( 'NONE', #19091, #1351, #4275 ) ;
#10951=ORIENTED_EDGE ( 'NONE', *, *, #9134, .T. ) ;
#10961=CARTESIAN_POINT ( 'NONE',  ( 79.78925230247502043, 142.5259582928263455, 20.00000000000000355 ) ) ;
#10967=DIRECTION ( 'NONE',  ( 0.000000000000000000, 0.000000000000000000, 1.000000000000000000 ) ) ;
#10968=CARTESIAN_POINT ( 'NONE',  ( 30.42502041961813575, 271.1055109169419097, -40.00000000000000000 ) ) ;
#10977=ORIENTED_EDGE ( 'NONE', *, *, #13147, .T. ) ;
#10989=ADVANCED_FACE ( 'NONE', ( #16013 ), #8961, .F. ) ;
#10994=DIRECTION ( 'NONE',  ( 0.000000000000000000, 1.000000000000000000, 0.000000000000000000 ) ) ;
#11004=EDGE_CURVE ( 'NONE', #12520, #12450, #3521, .T. ) ;
#11005=FACE_OUTER_BOUND ( 'NONE', #12495, .T. ) ;
#11007=EDGE_LOOP ( 'NONE', ( #2331, #5477, #1694, #7594, #3624, #10417 ) ) ;
#11029=ORIENTED_EDGE ( 'NONE', *, *, #20952, .F. ) ;
#11041=CARTESIAN_POINT ( 'NONE',  ( 6.416697501590670427, 217.7548513357008630, 60.00000000000000000 ) ) ;
#11047=DIRECTION ( 'NONE',  ( 0.000000000000000000, -1.000000000000000000, 0.000000000000000000 ) ) ;
#11057=ADVANCED_FACE ( 'NONE', ( #12861 ), #11437, .F. ) ;
#11067=PLANE ( 'NONE',  #20706 ) ;
#11073=CARTESIAN_POINT ( 'NONE',  ( -28.68588794268872633, 271.1055109169419666, -40.00000000000000000 ) ) ;
#11075=AXIS2_PLACEMENT_3D ( 'NONE', #6513, #6404, #1141 ) ;
#11076=CARTESIAN_POINT ( 'NONE',  ( 69.79185940953689737, 142.2976266388001250, 40.00000000000000000 ) ) ;
#11091=VECTOR ( 'NONE', #18275, 1000.000000000000000 ) ;
#11093=CARTESIAN_POINT ( 'NONE',  ( 107.6674317086782935, 187.4856410316723441, -20.00000000000000355 ) ) ;
#11098=LINE ( 'NONE', #13159, #10724 ) ;
#11103=DIRECTION ( 'NONE',  ( 1.000000000000000000, 0.000000000000000000, 0.000000000000000000 ) ) ;
#11120=ORIENTED_EDGE ( 'NONE', *, *, #10224, .F. ) ;
#11125=LINE ( 'NONE', #9609, #3 ) ;
#11137=EDGE_LOOP ( 'NONE', ( #12448, #20076, #14192, #6427 ) ) ;
#11140=ORIENTED_EDGE ( 'NONE', *, *, #15849, .T. ) ;
#11141=LINE ( 'NONE', #12985, #8009 ) ;
#11152=MANIFOLD_SOLID_BREP ( 'Cut-Extrude9', #728 ) ;
#11154=CARTESIAN_POINT ( 'NONE',  ( 60.03793209889851568, 30.52886280891152282, 136.1729372809869005 ) ) ;
#11157=EDGE_CURVE ( 'NONE', #15737, #8903, #6609, .T. ) ;
#11161=VECTOR ( 'NONE', #3252, 1000.000000000000000 ) ;
#11167=VERTEX_POINT ( 'NONE', #6250 ) ;
#11170=CARTESIAN_POINT ( 'NONE',  ( -33.23992160639906501, 53.12908672755433770, 49.39171662400100615 ) ) ;
#11179=DIRECTION ( 'NONE',  ( 0.000000000000000000, 1.000000000000000000, 0.000000000000000000 ) ) ;
#11180=VECTOR ( 'NONE', #11759, 1000.000000000000000 ) ;
#11182=CARTESIAN_POINT ( 'NONE',  ( -21.75104255857543478, 45.31773601326444378, 49.11655252816966311 ) ) ;
#11190=ADVANCED_FACE ( 'NONE', ( #11552 ), #7866, .F. ) ;
#11195=ORIENTED_EDGE ( 'NONE', *, *, #19817, .F. ) ;
#11196=LINE ( 'NONE', #4498, #1686 ) ;
#11197=ORIENTED_EDGE ( 'NONE', *, *, #17894, .F. ) ;
#11201=EDGE_CURVE ( 'NONE', #5985, #15324, #17825, .T. ) ;
#11202=EDGE_LOOP ( 'NONE', ( #21232, #12937, #765, #6215, #9170, #2503, #13262, #17968, #3200 ) ) ;
#11203=CARTESIAN_POINT ( 'NONE',  ( 6.416697501590670427, 172.9933428177121471, -50.00000000000000000 ) ) ;
#11205=EDGE_CURVE ( 'NONE', #13185, #16429, #11331, .T. ) ;
#11211=CARTESIAN_POINT ( 'NONE',  ( 0.000000000000000000, 31.85652257517428865, 0.000000000000000000 ) ) ;
#11214=DIRECTION ( 'NONE',  ( 0.000000000000000000, 1.000000000000000000, 0.000000000000000000 ) ) ;
#11226=EDGE_LOOP ( 'NONE', ( #2438, #8750, #20599, #21208 ) ) ;
#11242=ORIENTED_EDGE ( 'NONE', *, *, #7755, .T. ) ;
#11245=ORIENTED_EDGE ( 'NONE', *, *, #4332, .F. ) ;
#11254=PLANE ( 'NONE',  #14136 ) ;
#11263=LINE ( 'NONE', #15069, #4362 ) ;
#11264=EDGE_CURVE ( 'NONE', #17379, #11167, #18570, .T. ) ;
#11269=VECTOR ( 'NONE', #2955, 1000.000000000000000 ) ;
#11272=FACE_OUTER_BOUND ( 'NONE', #8537, .T. ) ;
#11277=EDGE_CURVE ( 'NONE', #15077, #4211, #19017, .T. ) ;
#11282=DIRECTION ( 'NONE',  ( 0.000000000000000000, 0.000000000000000000, 1.000000000000000000 ) ) ;
#11284=CARTESIAN_POINT ( 'NONE',  ( -20.19820727147837047, 45.49892208276283156, 48.87197369005792780 ) ) ;
#11287=DIRECTION ( 'NONE',  ( 0.9997392892938121722, 0.02283316540262222971, 0.000000000000000000 ) ) ;
#11289=AXIS2_PLACEMENT_3D ( 'NONE', #15440, #950, #12185 ) ;
#11300=VERTEX_POINT ( 'NONE', #10235 ) ;
#11304=VERTEX_POINT ( 'NONE', #12079 ) ;
#11307=ORIENTED_EDGE ( 'NONE', *, *, #8765, .T. ) ;
#11309=CARTESIAN_POINT ( 'NONE',  ( 68.91750629823305019, 180.5807618359183664, -53.41772401313671992 ) ) ;
#11329=ORIENTED_EDGE ( 'NONE', *, *, #21176, .F. ) ;
#11331=LINE ( 'NONE', #17926, #15624 ) ;
#11344=CARTESIAN_POINT ( 'NONE',  ( 2.416697501590669095, 217.7548513357008630, -49.99999999999999289 ) ) ;
#11351=ORIENTED_EDGE ( 'NONE', *, *, #18350, .F. ) ;
#11352=ORIENTED_EDGE ( 'NONE', *, *, #11004, .T. ) ;
#11353=FACE_OUTER_BOUND ( 'NONE', #15209, .T. ) ;
#11359=DIRECTION ( 'NONE',  ( 0.000000000000000000, 0.000000000000000000, -1.000000000000000000 ) ) ;
#11367=DIRECTION ( 'NONE',  ( 0.000000000000000000, 1.000000000000000000, 0.000000000000000000 ) ) ;
#11368=VECTOR ( 'NONE', #7819, 1000.000000000000000 ) ;
#11375=AXIS2_PLACEMENT_3D ( 'NONE', #20132, #2071, #245 ) ;
#11383=LINE ( 'NONE', #12702, #8645 ) ;
#11388=DIRECTION ( 'NONE',  ( -0.000000000000000000, -1.000000000000000000, -0.000000000000000000 ) ) ;
#11402=CARTESIAN_POINT ( 'NONE',  ( -123.2946569474810161, 10.52886280891152104, 20.57735571454641388 ) ) ;
#11407=DIRECTION ( 'NONE',  ( -0.000000000000000000, -0.000000000000000000, -1.000000000000000000 ) ) ;
#11411=DIRECTION ( 'NONE',  ( 0.000000000000000000, -1.000000000000000000, 0.000000000000000000 ) ) ;
#11412=EDGE_CURVE ( 'NONE', #9723, #12542, #3752, .T. ) ;
#11415=AXIS2_PLACEMENT_3D ( 'NONE', #20345, #5519, #12660 ) ;
#11416=DIRECTION ( 'NONE',  ( 0.000000000000000000, 0.000000000000000000, 1.000000000000000000 ) ) ;
#11420=FACE_OUTER_BOUND ( 'NONE', #20407, .T. ) ;
#11421=DIRECTION ( 'NONE',  ( 0.000000000000000000, 0.000000000000000000, -1.000000000000000000 ) ) ;
#11425=EDGE_CURVE ( 'NONE', #15685, #12221, #2042, .T. ) ;
#11426=LINE ( 'NONE', #6553, #2643 ) ;
#11428=CARTESIAN_POINT ( 'NONE',  ( 65.85920792673738333, 160.1716627696692683, -40.00000000000000000 ) ) ;
#11437=CYLINDRICAL_SURFACE ( 'NONE', #5925, 11.54039041455135184 ) ;
#11444=DIRECTION ( 'NONE',  ( -1.000000000000000000, 0.000000000000000000, 0.000000000000000000 ) ) ;
#11450=EDGE_CURVE ( 'NONE', #9674, #1161, #15238, .T. ) ;
#11455=ORIENTED_EDGE ( 'NONE', *, *, #9347, .F. ) ;
#11457=ORIENTED_EDGE ( 'NONE', *, *, #8372, .F. ) ;
#11473=LINE ( 'NONE', #11154, #12422 ) ;
#11476=AXIS2_PLACEMENT_3D ( 'NONE', #3637, #6765, #3736 ) ;
#11490=LINE ( 'NONE', #21125, #1084 ) ;
#11496=CARTESIAN_POINT ( 'NONE',  ( 81.24038404635966515, 56.85652257517428865, -94.99999999999994316 ) ) ;
#11502=CARTESIAN_POINT ( 'NONE',  ( -26.36169529657598076, 46.03899998623287360, 49.54893611991261793 ) ) ;
#11504=DIRECTION ( 'NONE',  ( 0.000000000000000000, -1.000000000000000000, 0.000000000000000000 ) ) ;
#11508=LINE ( 'NONE', #6414, #5072 ) ;
#11510=EDGE_CURVE ( 'NONE', #4211, #12773, #6016, .T. ) ;
#11519=ORIENTED_EDGE ( 'NONE', *, *, #13996, .F. ) ;
#11526=ORIENTED_EDGE ( 'NONE', *, *, #20326, .F. ) ;
#11528=CARTESIAN_POINT ( 'NONE',  ( -162.2727221670389781, 30.52886280891152282, 4.999999999999990230 ) ) ;
#11529=AXIS2_PLACEMENT_3D ( 'NONE', #2577, #5698, #15566 ) ;
#11538=CYLINDRICAL_SURFACE ( 'NONE', #11808, 4.000000000000001776 ) ;
#11539=CARTESIAN_POINT ( 'NONE',  ( 91.21585410611801592, 31.85652257517428865, 85.46735025547120301 ) ) ;
#11543=CARTESIAN_POINT ( 'NONE',  ( -10.76731745429009912, 50.09631838541057647, -118.3724535612433186 ) ) ;
#11549=CARTESIAN_POINT ( 'NONE',  ( 65.85920792673738333, 160.1716627696692683, 40.00000000000000000 ) ) ;
#11552=FACE_OUTER_BOUND ( 'NONE', #874, .T. ) ;
#11554=EDGE_LOOP ( 'NONE', ( #20499, #12077, #14514, #2459, #12648, #7991 ) ) ;
#11576=FACE_OUTER_BOUND ( 'NONE', #4048, .T. ) ;
#11592=DIRECTION ( 'NONE',  ( 0.000000000000000000, 1.000000000000000000, 0.000000000000000000 ) ) ;
#11593=EDGE_CURVE ( 'NONE', #16560, #5985, #13836, .T. ) ;
#11601=ADVANCED_FACE ( 'NONE', ( #12728 ), #21370, .T. ) ;
#11604=CARTESIAN_POINT ( 'NONE',  ( -49.57497958038186425, 230.5765313837437418, 60.00000000000000000 ) ) ;
#11612=CARTESIAN_POINT ( 'NONE',  ( -22.26996532928915329, 45.30456360475645283, 49.18697961254023454 ) ) ;
#11614=CARTESIAN_POINT ( 'NONE',  ( 28.16023193154655502, 323.8848358243226357, 20.00000000000000355 ) ) ;
#11622=DIRECTION ( 'NONE',  ( -0.000000000000000000, 1.000000000000000000, -0.000000000000000000 ) ) ;
#11626=ORIENTED_EDGE ( 'NONE', *, *, #3816, .F. ) ;
#11634=ORIENTED_EDGE ( 'NONE', *, *, #16104, .F. ) ;
#11636=CARTESIAN_POINT ( 'NONE',  ( -13.14633856003217360, 49.83395320290721031, -47.10416470750529783 ) ) ;
#11637=AXIS2_PLACEMENT_3D ( 'NONE', #3719, #4139, #703 ) ;
#11639=LINE ( 'NONE', #195, #11697 ) ;
#11641=PLANE ( 'NONE',  #19436 ) ;
#11655=VECTOR ( 'NONE', #12337, 1000.000000000000227 ) ;
#11656=EDGE_LOOP ( 'NONE', ( #9622, #14173, #8532 ) ) ;
#11658=EDGE_CURVE ( 'NONE', #13368, #10871, #3312, .T. ) ;
#11661=EDGE_LOOP ( 'NONE', ( #4603, #234, #9647, #9542, #4922 ) ) ;
#11663=FACE_OUTER_BOUND ( 'NONE', #17036, .T. ) ;
#11673=CARTESIAN_POINT ( 'NONE',  ( 20.42502041961813930, 230.5765313837437418, 60.00000000000000000 ) ) ;
#11681=VERTEX_POINT ( 'NONE', #8264 ) ;
#11691=ADVANCED_FACE ( 'NONE', ( #9474 ), #13044, .F. ) ;
#11693=CARTESIAN_POINT ( 'NONE',  ( 52.94681837068318941, 78.74778544605769071, 94.99999999999994316 ) ) ;
#11695=DIRECTION ( 'NONE',  ( 0.000000000000000000, 0.000000000000000000, 1.000000000000000000 ) ) ;
#11697=VECTOR ( 'NONE', #19750, 1000.000000000000000 ) ;
#11701=EDGE_CURVE ( 'NONE', #1447, #18698, #1082, .T. ) ;
#11709=CARTESIAN_POINT ( 'NONE',  ( 40.42502041961814996, 180.1716627696692967, -40.00000000000000000 ) ) ;
#11713=FACE_OUTER_BOUND ( 'NONE', #7222, .T. ) ;
#11720=DIRECTION ( 'NONE',  ( 0.000000000000000000, 0.000000000000000000, -1.000000000000000000 ) ) ;
#11728=VECTOR ( 'NONE', #9401, 1000.000000000000000 ) ;
#11735=EDGE_LOOP ( 'NONE', ( #7099, #11455 ) ) ;
#11737=ORIENTED_EDGE ( 'NONE', *, *, #2481, .F. ) ;
#11745=CARTESIAN_POINT ( 'NONE',  ( -25.36211449377851679, 45.71545155958810369, -49.49192749095595190 ) ) ;
#11756=CARTESIAN_POINT ( 'NONE',  ( -33.38097863509928942, 53.57231333527381878, -49.37834231071079927 ) ) ;
#11758=VERTEX_POINT ( 'NONE', #8486 ) ;
#11759=DIRECTION ( 'NONE',  ( 0.000000000000000000, -1.000000000000000000, 0.000000000000000000 ) ) ;
#11764=CARTESIAN_POINT ( 'NONE',  ( 20.42502041961813575, 271.1055109169419666, -20.00000000000000355 ) ) ;
#11780=ORIENTED_EDGE ( 'NONE', *, *, #18960, .T. ) ;
#11785=ORIENTED_EDGE ( 'NONE', *, *, #20411, .T. ) ;
#11790=AXIS2_PLACEMENT_3D ( 'NONE', #6911, #2065, #3777 ) ;
#11795=DIRECTION ( 'NONE',  ( 0.000000000000000000, -0.000000000000000000, 1.000000000000000000 ) ) ;
#11799=CARTESIAN_POINT ( 'NONE',  ( -31.66342138406952245, 50.08936347150523005, 120.9234288415484002 ) ) ;
#11806=VECTOR ( 'NONE', #7097, 1000.000000000000227 ) ;
#11807=ORIENTED_EDGE ( 'NONE', *, *, #16643, .T. ) ;
#11808=AXIS2_PLACEMENT_3D ( 'NONE', #10325, #6767, #3534 ) ;
#11811=EDGE_CURVE ( 'NONE', #10102, #6145, #19356, .T. ) ;
#11814=EDGE_LOOP ( 'NONE', ( #15074, #19243 ) ) ;
#11826=CARTESIAN_POINT ( 'NONE',  ( -22.30770786884145451, 56.85652257517428865, -152.3753892284480003 ) ) ;
#11832=LINE ( 'NONE', #281, #6935 ) ;
#11835=CARTESIAN_POINT ( 'NONE',  ( -24.91082379854346129, 45.60735762703961171, -122.4932255835355051 ) ) ;
#11839=VERTEX_POINT ( 'NONE', #11947 ) ;
#11847=CIRCLE ( 'NONE', #5277, 125.0000000000000000 ) ;
#11850=CARTESIAN_POINT ( 'NONE',  ( -26.35292120220072576, 46.04514432807761892, -49.54662401095963986 ) ) ;
#11852=DIRECTION ( 'NONE',  ( 0.000000000000000000, 0.000000000000000000, 1.000000000000000000 ) ) ;
#11856=AXIS2_PLACEMENT_3D ( 'NONE', #4409, #15778, #9481 ) ;
#11869=EDGE_CURVE ( 'NONE', #7807, #1524, #18856, .T. ) ;
#11870=CIRCLE ( 'NONE', #13613, 4.000000000000001776 ) ;
#11871=EDGE_CURVE ( 'NONE', #9392, #5108, #4046, .T. ) ;
#11872=ORIENTED_EDGE ( 'NONE', *, *, #107, .T. ) ;
#11879=ADVANCED_FACE ( 'NONE', ( #19083 ), #931, .T. ) ;
#11881=CARTESIAN_POINT ( 'NONE',  ( 88.28695088269886071, 152.5259582928263740, 20.00000000000000355 ) ) ;
#11901=DIRECTION ( 'NONE',  ( 0.000000000000000000, 1.000000000000000000, 0.000000000000000000 ) ) ;
#11905=CARTESIAN_POINT ( 'NONE',  ( -29.31767284124665807, 47.65796585322660661, 121.5149936206099284 ) ) ;
#11916=ORIENTED_EDGE ( 'NONE', *, *, #8627, .F. ) ;
#11929=CARTESIAN_POINT ( 'NONE',  ( 20.42502041961813575, 271.1055109169419666, -40.00000000000000000 ) ) ;
#11931=LINE ( 'NONE', #8360, #19015 ) ;
#11935=DIRECTION ( 'NONE',  ( -0.000000000000000000, -0.000000000000000000, 1.000000000000000000 ) ) ;
#11937=LINE ( 'NONE', #10733, #2318 ) ;
#11941=ORIENTED_EDGE ( 'NONE', *, *, #1569, .F. ) ;
#11946=ORIENTED_EDGE ( 'NONE', *, *, #18597, .F. ) ;
#11947=CARTESIAN_POINT ( 'NONE',  ( -22.30770786884143675, 45.31613216062291372, 122.9933582338429687 ) ) ;
#11949=VERTEX_POINT ( 'NONE', #7391 ) ;
#11951=CARTESIAN_POINT ( 'NONE',  ( -26.84078544385846143, 46.24045653294090386, -49.56718956592591496 ) ) ;
#11954=DIRECTION ( 'NONE',  ( 0.000000000000000000, 0.000000000000000000, 1.000000000000000000 ) ) ;
#11956=DIRECTION ( 'NONE',  ( -1.000000000000000000, 0.000000000000000000, 0.000000000000000000 ) ) ;
#11957=EDGE_CURVE ( 'NONE', #12829, #7636, #2447, .T. ) ;
#11958=AXIS2_PLACEMENT_3D ( 'NONE', #3926, #700, #2423 ) ;
#11959=PLANE ( 'NONE',  #17659 ) ;
#11966=ADVANCED_FACE ( 'NONE', ( #15744 ), #7497, .T. ) ;
#11990=CARTESIAN_POINT ( 'NONE',  ( 60.69669829156632090, 56.85652257517428865, 94.99999999999994316 ) ) ;
#11993=EDGE_CURVE ( 'NONE', #18701, #5552, #20819, .T. ) ;
#11997=VERTEX_POINT ( 'NONE', #16274 ) ;
#12003=ORIENTED_EDGE ( 'NONE', *, *, #12040, .T. ) ;
#12014=CARTESIAN_POINT ( 'NONE',  ( -33.84809828339280102, 56.85652257517428865, -152.3753892284480003 ) ) ;
#12017=VERTEX_POINT ( 'NONE', #9653 ) ;
#12021=ORIENTED_EDGE ( 'NONE', *, *, #1392, .T. ) ;
#12038=CARTESIAN_POINT ( 'NONE',  ( 43.53705524234220547, -133.1434774248255906, 96.62835994548002816 ) ) ;
#12040=EDGE_CURVE ( 'NONE', #8154, #16087, #11383, .T. ) ;
#12046=CIRCLE ( 'NONE', #2735, 20.00000000000000000 ) ;
#12056=VERTEX_POINT ( 'NONE', #11496 ) ;
#12058=CARTESIAN_POINT ( 'NONE',  ( -21.74034274139373224, 45.28293352602295130, -49.12345169421191571 ) ) ;
#12061=LINE ( 'NONE', #18550, #8539 ) ;
#12062=AXIS2_PLACEMENT_3D ( 'NONE', #4985, #1537, #18070 ) ;
#12065=CARTESIAN_POINT ( 'NONE',  ( -123.2946569474810161, 30.52886280891152282, 20.57735571454641388 ) ) ;
#12066=DIRECTION ( 'NONE',  ( -1.374938938973709817E-16, 1.000000000000000000, 0.000000000000000000 ) ) ;
#12072=ORIENTED_EDGE ( 'NONE', *, *, #14335, .T. ) ;
#12075=VECTOR ( 'NONE', #21000, 1000.000000000000000 ) ;
#12076=ADVANCED_FACE ( 'NONE', ( #8128 ), #16064, .F. ) ;
#12077=ORIENTED_EDGE ( 'NONE', *, *, #16235, .T. ) ;
#12079=CARTESIAN_POINT ( 'NONE',  ( 81.24038404635966515, 56.85652257517428865, 94.99999999999994316 ) ) ;
#12084=CARTESIAN_POINT ( 'NONE',  ( 20.42502041961813575, 271.1055109169419666, 20.00000000000000355 ) ) ;
#12107=CIRCLE ( 'NONE', #8302, 5.000000000000004441 ) ;
#12111=AXIS2_PLACEMENT_3D ( 'NONE', #4610, #11407, #18012 ) ;
#12114=CARTESIAN_POINT ( 'NONE',  ( 51.98438129372387806, -133.1434774248255906, -117.7249735956185219 ) ) ;
#12117=AXIS2_PLACEMENT_3D ( 'NONE', #19609, #19190, #9333 ) ;
#12129=ADVANCED_FACE ( 'NONE', ( #6088 ), #19293, .T. ) ;
#12150=CARTESIAN_POINT ( 'NONE',  ( 125.7989814974898053, 10.52886280891152104, 40.00000000000000000 ) ) ;
#12152=MECHANICAL_DESIGN_GEOMETRIC_PRESENTATION_REPRESENTATION('',(#14239),#15962);
#12155=CARTESIAN_POINT ( 'NONE',  ( -27.39255831251362139, 46.46955322709327163, -121.9637379996554216 ) ) ;
#12158=EDGE_LOOP ( 'NONE', ( #6248, #12021, #3854, #2401, #16936, #1521 ) ) ;
#12164=CARTESIAN_POINT ( 'NONE',  ( -10.76731745429009912, 50.09631838541057647, 118.3724535612433186 ) ) ;
#12165=DIRECTION ( 'NONE',  ( 9.855701800883827197E-17, -1.000000000000000000, 0.000000000000000000 ) ) ;
#12167=AXIS2_PLACEMENT_3D ( 'NONE', #4306, #15568, #4194 ) ;
#12171=LINE ( 'NONE', #1040, #12417 ) ;
#12174=DIRECTION ( 'NONE',  ( -0.000000000000000000, -0.000000000000000000, -1.000000000000000000 ) ) ;
#12179=DIRECTION ( 'NONE',  ( 0.000000000000000000, 0.9253149302858357794, -0.3791995250394160633 ) ) ;
#12183=CARTESIAN_POINT ( 'NONE',  ( 60.03793209889851568, 30.52886280891152282, -152.3753892284480003 ) ) ;
#12185=DIRECTION ( 'NONE',  ( 0.000000000000000000, -0.000000000000000000, -1.000000000000000000 ) ) ;
#12187=ORIENTED_EDGE ( 'NONE', *, *, #7343, .T. ) ;
#12190=ADVANCED_FACE ( 'NONE', ( #11713 ), #6620, .F. ) ;
#12191=VERTEX_POINT ( 'NONE', #13241 ) ;
#12199=DIRECTION ( 'NONE',  ( 1.000000000000000000, 0.000000000000000000, 0.000000000000000000 ) ) ;
#12202=DIRECTION ( 'NONE',  ( 0.000000000000000000, -1.000000000000000000, 0.000000000000000000 ) ) ;
#12207=DIRECTION ( 'NONE',  ( -1.000000000000000000, 0.000000000000000000, 0.000000000000000000 ) ) ;
#12208=VECTOR ( 'NONE', #19409, 1000.000000000000000 ) ;
#12214=ORIENTED_EDGE ( 'NONE', *, *, #18138, .F. ) ;
#12221=VERTEX_POINT ( 'NONE', #4242 ) ;
#12227=VECTOR ( 'NONE', #13203, 1000.000000000000000 ) ;
#12231=PLANE ( 'NONE',  #496 ) ;
#12236=DIRECTION ( 'NONE',  ( 0.000000000000000000, 0.000000000000000000, -1.000000000000000000 ) ) ;
#12239=ORIENTED_EDGE ( 'NONE', *, *, #21176, .T. ) ;
#12242=VECTOR ( 'NONE', #10392, 1000.000000000000000 ) ;
#12263=CARTESIAN_POINT ( 'NONE',  ( 65.85920792673738333, 160.1716627696692683, 40.00000000000000000 ) ) ;
#12266=ORIENTED_EDGE ( 'NONE', *, *, #9956, .T. ) ;
#12271=FACE_BOUND ( 'NONE', #5391, .T. ) ;
#12272=ADVANCED_FACE ( 'NONE', ( #19438, #14587 ), #6234, .F. ) ;
#12273=VECTOR ( 'NONE', #8, 1000.000000000000000 ) ;
#12274=CARTESIAN_POINT ( 'NONE',  ( -18.68588794268873698, 323.8848358243226357, -20.00000000000000355 ) ) ;
#12277=ORIENTED_EDGE ( 'NONE', *, *, #17868, .T. ) ;
#12279=CARTESIAN_POINT ( 'NONE',  ( 62.02695467647412642, 160.1716627696692683, 61.71700053422265597 ) ) ;
#12285=CARTESIAN_POINT ( 'NONE',  ( 51.98438129372387806, 56.85652257517428865, 94.99999999999994316 ) ) ;
#12291=CARTESIAN_POINT ( 'NONE',  ( 51.50493485826542184, 141.8799693780962912, -20.00000000000000355 ) ) ;
#12293=ORIENTED_EDGE ( 'NONE', *, *, #3720, .F. ) ;
#12295=ORIENTED_EDGE ( 'NONE', *, *, #4148, .F. ) ;
#12301=CARTESIAN_POINT ( 'NONE',  ( -28.68588794268872633, 174.3162933293988033, 20.00000000000000000 ) ) ;
#12307=CARTESIAN_POINT ( 'NONE',  ( 60.03793209889851568, 30.52886280891152282, -136.1729372809869005 ) ) ;
#12311=LINE ( 'NONE', #20640, #19228 ) ;
#12316=LINE ( 'NONE', #7654, #15050 ) ;
#12319=DIRECTION ( 'NONE',  ( -0.000000000000000000, -0.000000000000000000, -1.000000000000000000 ) ) ;
#12320=VERTEX_POINT ( 'NONE', #11539 ) ;
#12324=ORIENTED_EDGE ( 'NONE', *, *, #19928, .F. ) ;
#12326=ORIENTED_EDGE ( 'NONE', *, *, #8147, .T. ) ;
#12329=VECTOR ( 'NONE', #3617, 1000.000000000000000 ) ;
#12336=VECTOR ( 'NONE', #592, 1000.000000000000000 ) ;
#12337=DIRECTION ( 'NONE',  ( -0.1337298367054296222, 0.9910178256594273094, -0.000000000000000000 ) ) ;
#12345=ORIENTED_EDGE ( 'NONE', *, *, #9134, .F. ) ;
#12346=ORIENTED_EDGE ( 'NONE', *, *, #3113, .F. ) ;
#12350=EDGE_CURVE ( 'NONE', #3575, #3125, #18339, .T. ) ;
#12375=DIRECTION ( 'NONE',  ( 0.000000000000000000, 1.000000000000000000, 0.000000000000000000 ) ) ;
#12390=EDGE_CURVE ( 'NONE', #16401, #16623, #6551, .T. ) ;
#12392=AXIS2_PLACEMENT_3D ( 'NONE', #639, #17808, #17392 ) ;
#12395=CARTESIAN_POINT ( 'NONE',  ( 35.96497763894178945, 230.5765313837437418, -60.00000000000000000 ) ) ;
#12400=CARTESIAN_POINT ( 'NONE',  ( -18.68588794268873698, 281.1055109169419666, 40.00000000000000000 ) ) ;
#12407=ORIENTED_EDGE ( 'NONE', *, *, #5647, .T. ) ;
#12409=AXIS2_PLACEMENT_3D ( 'NONE', #11826, #10088, #15511 ) ;
#12411=LINE ( 'NONE', #20742, #5817 ) ;
#12417=VECTOR ( 'NONE', #13799, 1000.000000000000000 ) ;
#12422=VECTOR ( 'NONE', #6282, 1000.000000000000000 ) ;
#12424=FACE_OUTER_BOUND ( 'NONE', #11202, .T. ) ;
#12427=ORIENTED_EDGE ( 'NONE', *, *, #11871, .T. ) ;
#12430=VERTEX_POINT ( 'NONE', #14030 ) ;
#12435=ORIENTED_EDGE ( 'NONE', *, *, #11201, .F. ) ;
#12446=LINE ( 'NONE', #9932, #1155 ) ;
#12448=ORIENTED_EDGE ( 'NONE', *, *, #13913, .F. ) ;
#12450=VERTEX_POINT ( 'NONE', #15337 ) ;
#12452=ORIENTED_EDGE ( 'NONE', *, *, #16038, .T. ) ;
#12457=EDGE_CURVE ( 'NONE', #11839, #15497, #6982, .T. ) ;
#12477=ADVANCED_FACE ( 'NONE', ( #727 ), #11959, .T. ) ;
#12484=ORIENTED_EDGE ( 'NONE', *, *, #12533, .F. ) ;
#12493=CARTESIAN_POINT ( 'NONE',  ( 27.98965548446208729, 333.8848358243226357, 40.00000000000000000 ) ) ;
#12495=EDGE_LOOP ( 'NONE', ( #10528, #17116, #8509, #9070, #216 ) ) ;
#12499=CARTESIAN_POINT ( 'NONE',  ( -18.68588794268873698, 323.8848358243226357, -40.00000000000000000 ) ) ;
#12501=DIRECTION ( 'NONE',  ( -9.855701800883827197E-17, 1.000000000000000000, -0.000000000000000000 ) ) ;
#12502=CARTESIAN_POINT ( 'NONE',  ( 10.41669750159067220, 217.7548513357008630, 49.99999999999999289 ) ) ;
#12503=CARTESIAN_POINT ( 'NONE',  ( -33.84809828339280102, 56.85652257517428865, 120.3299889578561448 ) ) ;
#12514=ORIENTED_EDGE ( 'NONE', *, *, #16643, .F. ) ;
#12520=VERTEX_POINT ( 'NONE', #2449 ) ;
#12521=DIRECTION ( 'NONE',  ( -1.000000000000000000, 0.000000000000000000, 0.000000000000000000 ) ) ;
#12522=CARTESIAN_POINT ( 'NONE',  ( 115.7989814974898337, 142.5259582928263455, -20.00000000000000355 ) ) ;
#12533=EDGE_CURVE ( 'NONE', #5288, #1858, #20610, .T. ) ;
#12536=EDGE_CURVE ( 'NONE', #20892, #795, #14557, .T. ) ;
#12540=AXIS2_PLACEMENT_3D ( 'NONE', #835, #7401, #14555 ) ;
#12542=VERTEX_POINT ( 'NONE', #15653 ) ;
#12544=ORIENTED_EDGE ( 'NONE', *, *, #12457, .F. ) ;
#12548=ORIENTED_EDGE ( 'NONE', *, *, #7052, .T. ) ;
#12551=ORIENTED_EDGE ( 'NONE', *, *, #13411, .F. ) ;
#12563=DIRECTION ( 'NONE',  ( 0.000000000000000000, -1.000000000000000000, 0.000000000000000000 ) ) ;
#12565=ORIENTED_EDGE ( 'NONE', *, *, #1574, .F. ) ;
#12568=ORIENTED_EDGE ( 'NONE', *, *, #8275, .T. ) ;
#12572=VECTOR ( 'NONE', #12501, 1000.000000000000000 ) ;
#12587=ADVANCED_FACE ( 'NONE', ( #3848 ), #4060, .T. ) ;
#12606=EDGE_CURVE ( 'NONE', #17381, #952, #15756, .T. ) ;
#12608=FACE_OUTER_BOUND ( 'NONE', #8157, .T. ) ;
#12610=CARTESIAN_POINT ( 'NONE',  ( 105.7989814974898479, 142.5259582928263455, -40.00000000000000000 ) ) ;
#12619=ORIENTED_EDGE ( 'NONE', *, *, #4848, .T. ) ;
#12620=ORIENTED_EDGE ( 'NONE', *, *, #6973, .F. ) ;
#12621=CARTESIAN_POINT ( 'NONE',  ( 6.416697501590670427, 172.9933428177121471, 60.00000000000000000 ) ) ;
#12625=DIRECTION ( 'NONE',  ( 0.9999562017632421806, 0.000000000000000000, -0.009359196291876339252 ) ) ;
#12636=FACE_OUTER_BOUND ( 'NONE', #13636, .T. ) ;
#12639=EDGE_CURVE ( 'NONE', #17724, #264, #13602, .T. ) ;
#12640=CARTESIAN_POINT ( 'NONE',  ( -49.57497958038186425, 230.5765313837437418, 49.99999999999999289 ) ) ;
#12646=CARTESIAN_POINT ( 'NONE',  ( 105.7989814974898479, 152.5259582928263740, -40.00000000000000000 ) ) ;
#12647=ORIENTED_EDGE ( 'NONE', *, *, #19479, .F. ) ;
#12648=ORIENTED_EDGE ( 'NONE', *, *, #19987, .T. ) ;
#12658=AXIS2_PLACEMENT_3D ( 'NONE', #16364, #21227, #18078 ) ;
#12659=DIRECTION ( 'NONE',  ( -1.000000000000000000, 0.000000000000000000, 0.000000000000000000 ) ) ;
#12660=DIRECTION ( 'NONE',  ( 1.000000000000000000, 0.000000000000000000, 0.000000000000000000 ) ) ;
#12666=ORIENTED_EDGE ( 'NONE', *, *, #17545, .F. ) ;
#12682=CARTESIAN_POINT ( 'NONE',  ( 35.96497763894178945, 230.5765313837437418, -40.00000000000000000 ) ) ;
#12688=AXIS2_PLACEMENT_3D ( 'NONE', #8467, #8247, #19837 ) ;
#12693=AXIS2_PLACEMENT_3D ( 'NONE', #17001, #18604, #8550 ) ;
#12697=VERTEX_POINT ( 'NONE', #4493 ) ;
#12702=CARTESIAN_POINT ( 'NONE',  ( 20.42502041961813930, 230.5765313837437418, 60.00000000000000000 ) ) ;
#12712=CARTESIAN_POINT ( 'NONE',  ( 72.94945500224395118, 285.0140030772282103, -40.00000000000000000 ) ) ;
#12713=PLANE ( 'NONE',  #6442 ) ;
#12723=DIRECTION ( 'NONE',  ( 0.000000000000000000, 0.000000000000000000, 1.000000000000000000 ) ) ;
#12724=ORIENTED_EDGE ( 'NONE', *, *, #8275, .F. ) ;
#12728=FACE_OUTER_BOUND ( 'NONE', #6478, .T. ) ;
#12731=DIRECTION ( 'NONE',  ( 0.000000000000000000, 0.000000000000000000, -1.000000000000000000 ) ) ;
#12734=LINE ( 'NONE', #19325, #15169 ) ;
#12750=VECTOR ( 'NONE', #17022, 1000.000000000000000 ) ;
#12755=LINE ( 'NONE', #9285, #16302 ) ;
#12765=CIRCLE ( 'NONE', #7213, 10.00000000000000533 ) ;
#12768=FACE_OUTER_BOUND ( 'NONE', #1414, .T. ) ;
#12770=LINE ( 'NONE', #21303, #12273 ) ;
#12773=VERTEX_POINT ( 'NONE', #7726 ) ;
#12780=CYLINDRICAL_SURFACE ( 'NONE', #3824, 28.29169339157297358 ) ;
#12783=DIRECTION ( 'NONE',  ( 1.000000000000000000, -0.000000000000000000, 0.000000000000000000 ) ) ;
#12784=EDGE_CURVE ( 'NONE', #14197, #7633, #10865, .T. ) ;
#12790=LINE ( 'NONE', #5753, #5761 ) ;
#12794=AXIS2_PLACEMENT_3D ( 'NONE', #808, #2419, #696 ) ;
#12802=DIRECTION ( 'NONE',  ( 1.000000000000000000, 0.000000000000000000, 0.000000000000000000 ) ) ;
#12803=VERTEX_POINT ( 'NONE', #16292 ) ;
#12804=DIRECTION ( 'NONE',  ( 0.000000000000000000, -1.000000000000000000, 0.000000000000000000 ) ) ;
#12809=ORIENTED_EDGE ( 'NONE', *, *, #4721, .T. ) ;
#12810=VECTOR ( 'NONE', #3100, 1000.000000000000000 ) ;
#12814=EDGE_CURVE ( 'NONE', #11997, #12017, #19622, .T. ) ;
#12821=CARTESIAN_POINT ( 'NONE',  ( 10.41669750159067220, 172.9933428177121471, 50.00000000000000000 ) ) ;
#12826=DIRECTION ( 'NONE',  ( 0.000000000000000000, -1.000000000000000000, 0.000000000000000000 ) ) ;
#12828=ORIENTED_EDGE ( 'NONE', *, *, #16551, .F. ) ;
#12829=VERTEX_POINT ( 'NONE', #13142 ) ;
#12840=DIRECTION ( 'NONE',  ( 0.000000000000000000, 1.000000000000000000, 0.000000000000000000 ) ) ;
#12861=FACE_OUTER_BOUND ( 'NONE', #7089, .T. ) ;
#12877=LINE ( 'NONE', #17941, #17386 ) ;
#12879=EDGE_CURVE ( 'NONE', #5562, #14726, #18843, .T. ) ;
#12881=CYLINDRICAL_SURFACE ( 'NONE', #17749, 4.000000000000001776 ) ;
#12885=ORIENTED_EDGE ( 'NONE', *, *, #11201, .T. ) ;
#12889=PLANE ( 'NONE',  #1795 ) ;
#12893=FACE_OUTER_BOUND ( 'NONE', #21205, .T. ) ;
#12901=DIRECTION ( 'NONE',  ( 0.000000000000000000, 1.000000000000000000, 0.000000000000000000 ) ) ;
#12902=DIRECTION ( 'NONE',  ( 0.000000000000000000, 0.000000000000000000, -1.000000000000000000 ) ) ;
#12906=AXIS2_PLACEMENT_3D ( 'NONE', #4880, #18072, #11695 ) ;
#12920=CARTESIAN_POINT ( 'NONE',  ( 28.16023193154655502, 323.8848358243226357, -40.00000000000000000 ) ) ;
#12922=CARTESIAN_POINT ( 'NONE',  ( -28.24026808052491688, 46.95427799011174841, 49.59944287259298790 ) ) ;
#12923=DIRECTION ( 'NONE',  ( -0.000000000000000000, -1.000000000000000000, -0.000000000000000000 ) ) ;
#12926=EDGE_CURVE ( 'NONE', #16401, #5562, #13783, .T. ) ;
#12927=AXIS2_PLACEMENT_3D ( 'NONE', #17193, #2587, #8845 ) ;
#12935=EDGE_CURVE ( 'NONE', #10361, #9753, #17489, .T. ) ;
#12936=ORIENTED_EDGE ( 'NONE', *, *, #19928, .T. ) ;
#12937=ORIENTED_EDGE ( 'NONE', *, *, #15923, .T. ) ;
#12942=ORIENTED_EDGE ( 'NONE', *, *, #10887, .F. ) ;
#12947=CARTESIAN_POINT ( 'NONE',  ( 0.000000000000000000, 10.52886280891152104, 0.000000000000000000 ) ) ;
#12956=LINE ( 'NONE', #3114, #10916 ) ;
#12964=CARTESIAN_POINT ( 'NONE',  ( 115.7989814974898337, 152.5259582928263740, 40.00000000000000000 ) ) ;
#12966=VERTEX_POINT ( 'NONE', #387 ) ;
#12982=ORIENTED_EDGE ( 'NONE', *, *, #13913, .T. ) ;
#12985=CARTESIAN_POINT ( 'NONE',  ( 51.98438129372387806, -133.1434774248255906, -94.99999999999994316 ) ) ;
#12987=CARTESIAN_POINT ( 'NONE',  ( 118.4271928232701043, 31.85652257517428865, 40.00000000000000711 ) ) ;
#12993=ADVANCED_FACE ( 'NONE', ( #8686 ), #5334, .F. ) ;
#12994=VECTOR ( 'NONE', #11047, 1000.000000000000000 ) ;
#13011=DIRECTION ( 'NONE',  ( 0.000000000000000000, -1.000000000000000000, 0.000000000000000000 ) ) ;
#13012=ORIENTED_EDGE ( 'NONE', *, *, #16425, .T. ) ;
#13013=CARTESIAN_POINT ( 'NONE',  ( -29.48036301152122718, 47.76573509908928372, 49.60091809715360966 ) ) ;
#13016=PLANE ( 'NONE',  #12117 ) ;
#13017=CARTESIAN_POINT ( 'NONE',  ( 65.85920792673738333, 160.1716627696692683, 40.00000000000000000 ) ) ;
#13021=EDGE_CURVE ( 'NONE', #17195, #19655, #16821, .T. ) ;
#13023=CARTESIAN_POINT ( 'NONE',  ( -12.95795174569926722, 50.01372181642471304, 47.04466289070994378 ) ) ;
#13030=CARTESIAN_POINT ( 'NONE',  ( -123.2946569474810303, 10.52886280891152104, -20.57735571454641388 ) ) ;
#13033=AXIS2_PLACEMENT_3D ( 'NONE', #19156, #7673, #12659 ) ;
#13042=AXIS2_PLACEMENT_3D ( 'NONE', #1926, #5254, #8493 ) ;
#13043=ORIENTED_EDGE ( 'NONE', *, *, #15071, .T. ) ;
#13044=CYLINDRICAL_SURFACE ( 'NONE', #12111, 43.46661168214937732 ) ;
#13056=DIRECTION ( 'NONE',  ( 0.000000000000000000, 0.000000000000000000, -1.000000000000000000 ) ) ;
#13059=CARTESIAN_POINT ( 'NONE',  ( 40.42502041961814996, 170.1716627696692683, 40.00000000000000000 ) ) ;
#13066=EDGE_CURVE ( 'NONE', #15561, #19827, #17029, .T. ) ;
#13069=EDGE_CURVE ( 'NONE', #15822, #11300, #2317, .T. ) ;
#13071=ORIENTED_EDGE ( 'NONE', *, *, #8287, .T. ) ;
#13073=DIRECTION ( 'NONE',  ( -0.000000000000000000, -0.000000000000000000, 1.000000000000000000 ) ) ;
#13082=CARTESIAN_POINT ( 'NONE',  ( -22.30770786884145451, 30.52886280891152282, 122.9933582338429972 ) ) ;
#13097=FACE_BOUND ( 'NONE', #16771, .T. ) ;
#13101=EDGE_CURVE ( 'NONE', #13316, #15497, #19385, .T. ) ;
#13104=DIRECTION ( 'NONE',  ( 0.000000000000000000, -1.000000000000000000, 0.000000000000000000 ) ) ;
#13106=AXIS2_PLACEMENT_3D ( 'NONE', #2737, #4025, #9211 ) ;
#13110=DIRECTION ( 'NONE',  ( 0.000000000000000000, 0.000000000000000000, -1.000000000000000000 ) ) ;
#13112=DIRECTION ( 'NONE',  ( -0.000000000000000000, 1.000000000000000000, -0.000000000000000000 ) ) ;
#13113=CARTESIAN_POINT ( 'NONE',  ( 20.42502041961813930, 230.5765313837437418, 40.00000000000000000 ) ) ;
#13118=ORIENTED_EDGE ( 'NONE', *, *, #20988, .F. ) ;
#13122=EDGE_CURVE ( 'NONE', #4584, #7636, #4356, .T. ) ;
#13123=ORIENTED_EDGE ( 'NONE', *, *, #11412, .F. ) ;
#13125=ORIENTED_EDGE ( 'NONE', *, *, #8950, .F. ) ;
#13126=CARTESIAN_POINT ( 'NONE',  ( -31.45575705393271448, 49.80536212050644451, 49.52427915835843208 ) ) ;
#13134=CARTESIAN_POINT ( 'NONE',  ( 43.53705524234220547, 56.85652257517428865, 96.62835994548002816 ) ) ;
#13135=FACE_OUTER_BOUND ( 'NONE', #11226, .T. ) ;
#13141=CARTESIAN_POINT ( 'NONE',  ( 35.96497763894178945, 230.5765313837437418, 40.00000000000000000 ) ) ;
#13142=CARTESIAN_POINT ( 'NONE',  ( -22.30770786884145451, 10.52886280891152104, 122.9933582338429972 ) ) ;
#13147=EDGE_CURVE ( 'NONE', #13610, #2785, #4570, .T. ) ;
#13155=DIRECTION ( 'NONE',  ( 0.000000000000000000, 0.000000000000000000, -1.000000000000000000 ) ) ;
#13159=CARTESIAN_POINT ( 'NONE',  ( 2.416697501590669095, 172.9933428177121471, -45.00000000000000000 ) ) ;
#13160=VECTOR ( 'NONE', #3205, 1000.000000000000000 ) ;
#13162=AXIS2_PLACEMENT_3D ( 'NONE', #6398, #13011, #4780 ) ;
#13166=CIRCLE ( 'NONE', #15240, 53.46661168214943416 ) ;
#13169=CARTESIAN_POINT ( 'NONE',  ( 51.50493485826542184, 141.8799693780962912, -94.99999999999994316 ) ) ;
#13180=DIRECTION ( 'NONE',  ( -1.000000000000000000, 0.000000000000000000, -8.901024030850960568E-17 ) ) ;
#13185=VERTEX_POINT ( 'NONE', #6183 ) ;
#13187=CARTESIAN_POINT ( 'NONE',  ( 60.03793209889851568, 30.52886280891152282, 131.1729372809869005 ) ) ;
#13193=AXIS2_PLACEMENT_3D ( 'NONE', #5715, #10684, #15584 ) ;
#13194=DIRECTION ( 'NONE',  ( 0.000000000000000000, 1.000000000000000000, 0.000000000000000000 ) ) ;
#13203=DIRECTION ( 'NONE',  ( 1.000000000000000000, 1.250996701150283068E-16, -0.000000000000000000 ) ) ;
#13206=ADVANCED_FACE ( 'NONE', ( #9216 ), #2850, .F. ) ;
#13207=ORIENTED_EDGE ( 'NONE', *, *, #11450, .F. ) ;
#13211=DIRECTION ( 'NONE',  ( -0.000000000000000000, 1.000000000000000000, -0.000000000000000000 ) ) ;
#13217=CYLINDRICAL_SURFACE ( 'NONE', #8224, 20.57735571454641033 ) ;
#13223=CIRCLE ( 'NONE', #12540, 4.000000000000001776 ) ;
#13237=LINE ( 'NONE', #11604, #1199 ) ;
#13241=CARTESIAN_POINT ( 'NONE',  ( 20.42502041961815351, 163.4113008177049551, 60.00000000000000000 ) ) ;
#13249=DIRECTION ( 'NONE',  ( 0.000000000000000000, -1.000000000000000000, 0.000000000000000000 ) ) ;
#13250=DIRECTION ( 'NONE',  ( 0.000000000000000000, 0.000000000000000000, 1.000000000000000000 ) ) ;
#13252=EDGE_CURVE ( 'NONE', #15047, #6356, #14532, .T. ) ;
#13255=DIRECTION ( 'NONE',  ( 0.000000000000000000, 1.000000000000000000, 0.000000000000000000 ) ) ;
#13258=CYLINDRICAL_SURFACE ( 'NONE', #6793, 49.60091809715359545 ) ;
#13262=ORIENTED_EDGE ( 'NONE', *, *, #595, .T. ) ;
#13271=ORIENTED_EDGE ( 'NONE', *, *, #4990, .F. ) ;
#13274=VECTOR ( 'NONE', #7326, 1000.000000000000000 ) ;
#13288=AXIS2_PLACEMENT_3D ( 'NONE', #15182, #8880, #16802 ) ;
#13291=EDGE_CURVE ( 'NONE', #1447, #15711, #9533, .T. ) ;
#13302=CARTESIAN_POINT ( 'NONE',  ( 0.000000000000000000, 10.52886280891152104, 0.000000000000000000 ) ) ;
#13316=VERTEX_POINT ( 'NONE', #4463 ) ;
#13334=CARTESIAN_POINT ( 'NONE',  ( 20.42502041961813575, 271.1055109169419666, 40.00000000000000000 ) ) ;
#13343=DIRECTION ( 'NONE',  ( 1.000000000000000000, 9.855701800883827197E-17, -0.000000000000000000 ) ) ;
#13352=CYLINDRICAL_SURFACE ( 'NONE', #19008, 43.46661168214937732 ) ;
#13354=LINE ( 'NONE', #19943, #13789 ) ;
#13355=PLANE ( 'NONE',  #16153 ) ;
#13356=DIRECTION ( 'NONE',  ( 0.000000000000000000, 0.000000000000000000, 1.000000000000000000 ) ) ;
#13367=VECTOR ( 'NONE', #16639, 1000.000000000000000 ) ;
#13368=VERTEX_POINT ( 'NONE', #8226 ) ;
#13373=ORIENTED_EDGE ( 'NONE', *, *, #8116, .T. ) ;
#13378=CARTESIAN_POINT ( 'NONE',  ( -19.45117422794473683, 45.67224592879905742, -48.73435233020793333 ) ) ;
#13383=DIRECTION ( 'NONE',  ( 1.000000000000000000, 0.000000000000000000, 0.000000000000000000 ) ) ;
#13385=PLANE ( 'NONE',  #21169 ) ;
#13395=CIRCLE ( 'NONE', #6809, 4.000000000000001776 ) ;
#13403=ORIENTED_EDGE ( 'NONE', *, *, #14210, .T. ) ;
#13411=EDGE_CURVE ( 'NONE', #4398, #2785, #11263, .T. ) ;
#13419=ORIENTED_EDGE ( 'NONE', *, *, #179, .F. ) ;
#13420=ORIENTED_EDGE ( 'NONE', *, *, #8952, .T. ) ;
#13434=AXIS2_PLACEMENT_3D ( 'NONE', #9673, #9468, #1259 ) ;
#13435=CARTESIAN_POINT ( 'NONE',  ( -32.65721457343089185, 51.69451264534966128, 120.6590201788547319 ) ) ;
#13447=FACE_OUTER_BOUND ( 'NONE', #7738, .T. ) ;
#13471=LINE ( 'NONE', #18108, #15788 ) ;
#13476=ORIENTED_EDGE ( 'NONE', *, *, #18138, .T. ) ;
#13479=ADVANCED_FACE ( 'NONE', ( #3272 ), #6718, .F. ) ;
#13483=VERTEX_POINT ( 'NONE', #30 ) ;
#13490=DIRECTION ( 'NONE',  ( 0.000000000000000000, 1.000000000000000000, 0.000000000000000000 ) ) ;
#13495=AXIS2_PLACEMENT_3D ( 'NONE', #16811, #4904, #18310 ) ;
#13499=DIRECTION ( 'NONE',  ( 0.000000000000000000, 0.000000000000000000, 1.000000000000000000 ) ) ;
#13501=ORIENTED_EDGE ( 'NONE', *, *, #7194, .T. ) ;
#13509=VECTOR ( 'NONE', #15398, 1000.000000000000114 ) ;
#13525=ORIENTED_EDGE ( 'NONE', *, *, #2353, .T. ) ;
#13529=LINE ( 'NONE', #1634, #11161 ) ;
#13530=ORIENTED_EDGE ( 'NONE', *, *, #11701, .T. ) ;
#13544=DIRECTION ( 'NONE',  ( -0.000000000000000000, -0.000000000000000000, 1.000000000000000000 ) ) ;
#13546=EDGE_CURVE ( 'NONE', #8292, #7438, #6392, .T. ) ;
#13577=CARTESIAN_POINT ( 'NONE',  ( 69.79185940953689737, 142.2976266388001250, -69.11456258820064136 ) ) ;
#13585=ORIENTED_EDGE ( 'NONE', *, *, #7810, .T. ) ;
#13593=ORIENTED_EDGE ( 'NONE', *, *, #2446, .T. ) ;
#13602=LINE ( 'NONE', #5575, #10730 ) ;
#13610=VERTEX_POINT ( 'NONE', #14165 ) ;
#13611=CARTESIAN_POINT ( 'NONE',  ( -162.2727221670389781, 30.52886280891152282, 0.000000000000000000 ) ) ;
#13613=AXIS2_PLACEMENT_3D ( 'NONE', #16361, #13544, #21323 ) ;
#13618=ORIENTED_EDGE ( 'NONE', *, *, #5178, .F. ) ;
#13620=DIRECTION ( 'NONE',  ( -0.000000000000000000, -0.000000000000000000, 1.000000000000000000 ) ) ;
#13626=AXIS2_PLACEMENT_3D ( 'NONE', #18479, #3456, #8312 ) ;
#13628=LINE ( 'NONE', #2264, #5441 ) ;
#13634=CYLINDRICAL_SURFACE ( 'NONE', #3573, 220.7252770684331438 ) ;
#13636=EDGE_LOOP ( 'NONE', ( #1917, #5138, #20466 ) ) ;
#13639=CARTESIAN_POINT ( 'NONE',  ( -33.84809828339280102, 56.85652257517428865, -152.3753892284480003 ) ) ;
#13651=CARTESIAN_POINT ( 'NONE',  ( -23.81512245425836838, 45.39025379435859975, 122.7127025493173846 ) ) ;
#13660=ORIENTED_EDGE ( 'NONE', *, *, #7414, .T. ) ;
#13675=LINE ( 'NONE', #3713, #12336 ) ;
#13683=ORIENTED_EDGE ( 'NONE', *, *, #595, .F. ) ;
#13685=VERTEX_POINT ( 'NONE', #3585 ) ;
#13687=CARTESIAN_POINT ( 'NONE',  ( 28.16023193154655502, 323.8848358243226357, 20.00000000000000355 ) ) ;
#13689=DIRECTION ( 'NONE',  ( 0.000000000000000000, 0.000000000000000000, -1.000000000000000000 ) ) ;
#13696=CARTESIAN_POINT ( 'NONE',  ( 51.98438129372387806, -133.1434774248255906, 117.7249735956185219 ) ) ;
#13699=CARTESIAN_POINT ( 'NONE',  ( 115.7989814974898337, 142.5259582928263455, 20.00000000000000355 ) ) ;
#13703=DIRECTION ( 'NONE',  ( -0.000000000000000000, -1.000000000000000000, -0.000000000000000000 ) ) ;
#13714=VERTEX_POINT ( 'NONE', #8069 ) ;
#13722=AXIS2_PLACEMENT_3D ( 'NONE', #11076, #9132, #15754 ) ;
#13730=EDGE_CURVE ( 'NONE', #952, #10871, #16122, .T. ) ;
#13732=CARTESIAN_POINT ( 'NONE',  ( -162.2727221670389781, 10.52886280891152104, 0.000000000000000000 ) ) ;
#13734=ADVANCED_FACE ( 'NONE', ( #3116 ), #14699, .T. ) ;
#13740=ORIENTED_EDGE ( 'NONE', *, *, #9485, .T. ) ;
#13747=ADVANCED_FACE ( 'NONE', ( #9800 ), #16423, .F. ) ;
#13753=DIRECTION ( 'NONE',  ( -1.000000000000000000, 0.000000000000000000, 0.000000000000000000 ) ) ;
#13755=FACE_OUTER_BOUND ( 'NONE', #572, .T. ) ;
#13763=ORIENTED_EDGE ( 'NONE', *, *, #9152, .T. ) ;
#13783=LINE ( 'NONE', #16926, #2302 ) ;
#13786=CARTESIAN_POINT ( 'NONE',  ( -32.27528734226235230, 51.02792179363947156, -120.7615045227926771 ) ) ;
#13789=VECTOR ( 'NONE', #20366, 1000.000000000000000 ) ;
#13792=ORIENTED_EDGE ( 'NONE', *, *, #6044, .F. ) ;
#13799=DIRECTION ( 'NONE',  ( -0.000000000000000000, -0.000000000000000000, -1.000000000000000000 ) ) ;
#13800=EDGE_CURVE ( 'NONE', #13714, #9575, #9559, .T. ) ;
#13802=PLANE ( 'NONE',  #7560 ) ;
#13817=VERTEX_POINT ( 'NONE', #14382 ) ;
#13824=ORIENTED_EDGE ( 'NONE', *, *, #12784, .T. ) ;
#13834=DIRECTION ( 'NONE',  ( 1.000000000000000000, 0.000000000000000000, 0.000000000000000000 ) ) ;
#13836=CIRCLE ( 'NONE', #4510, 9.999999999999994671 ) ;
#13847=VECTOR ( 'NONE', #1480, 1000.000000000000000 ) ;
#13856=ADVANCED_FACE ( 'NONE', ( #15128 ), #5048, .F. ) ;
#13867=EDGE_CURVE ( 'NONE', #4551, #13714, #1518, .T. ) ;
#13870=VERTEX_POINT ( 'NONE', #8502 ) ;
#13875=LINE ( 'NONE', #20464, #20165 ) ;
#13888=LINE ( 'NONE', #2203, #12750 ) ;
#13892=LINE ( 'NONE', #8794, #7632 ) ;
#13913=EDGE_CURVE ( 'NONE', #4442, #534, #2656, .T. ) ;
#13917=DIRECTION ( 'NONE',  ( 0.000000000000000000, -1.000000000000000000, 0.000000000000000000 ) ) ;
#13919=CARTESIAN_POINT ( 'NONE',  ( 43.53705524234220547, 30.52886280891152282, 96.62835994548002816 ) ) ;
#13923=VECTOR ( 'NONE', #11287, 999.9999999999998863 ) ;
#13935=ORIENTED_EDGE ( 'NONE', *, *, #18002, .T. ) ;
#13938=VECTOR ( 'NONE', #12236, 1000.000000000000000 ) ;
#13944=CARTESIAN_POINT ( 'NONE',  ( 51.50493485826542184, 170.1716627696692683, 57.52045949366692668 ) ) ;
#13951=PLANE ( 'NONE',  #6786 ) ;
#13965=ORIENTED_EDGE ( 'NONE', *, *, #6044, .T. ) ;
#13966=EDGE_CURVE ( 'NONE', #6673, #9723, #18154, .T. ) ;
#13967=AXIS2_PLACEMENT_3D ( 'NONE', #17354, #928, #1138 ) ;
#13981=ORIENTED_EDGE ( 'NONE', *, *, #10224, .T. ) ;
#13987=ORIENTED_EDGE ( 'NONE', *, *, #8517, .F. ) ;
#13988=ORIENTED_EDGE ( 'NONE', *, *, #9568, .T. ) ;
#13996=EDGE_CURVE ( 'NONE', #15047, #9674, #9035, .T. ) ;
#14002=( NAMED_UNIT ( * ) PLANE_ANGLE_UNIT ( ) SI_UNIT ( $, .RADIAN. ) );
#14005=DIRECTION ( 'NONE',  ( -0.3717199501173604759, 0.000000000000000000, -0.9283449136418786551 ) ) ;
#14006=CARTESIAN_POINT ( 'NONE',  ( 0.000000000000000000, 10.52886280891152104, 0.000000000000000000 ) ) ;
#14017=LINE ( 'NONE', #18968, #17631 ) ;
#14018=CARTESIAN_POINT ( 'NONE',  ( 0.000000000000000000, 10.52886280891152104, 0.000000000000000000 ) ) ;
#14020=ORIENTED_EDGE ( 'NONE', *, *, #10803, .F. ) ;
#14025=CARTESIAN_POINT ( 'NONE',  ( -28.68588794268874054, 333.8848358243226357, -40.00000000000000000 ) ) ;
#14030=CARTESIAN_POINT ( 'NONE',  ( 88.28695088269886071, 142.5259582928263455, -20.00000000000000355 ) ) ;
#14044=EDGE_LOOP ( 'NONE', ( #4678, #17842, #20492, #12324 ) ) ;
#14047=DIRECTION ( 'NONE',  ( 0.000000000000000000, 1.000000000000000000, 0.000000000000000000 ) ) ;
#14048=CARTESIAN_POINT ( 'NONE',  ( 6.416697501590670427, 217.7548513357008630, -60.00000000000000000 ) ) ;
#14055=DIRECTION ( 'NONE',  ( 0.000000000000000000, 1.000000000000000000, 0.000000000000000000 ) ) ;
#14062=ORIENTED_EDGE ( 'NONE', *, *, #6785, .T. ) ;
#14067=CARTESIAN_POINT ( 'NONE',  ( 30.42502041961814996, 170.1716627696692683, -20.00000000000000355 ) ) ;
#14078=DIRECTION ( 'NONE',  ( 0.000000000000000000, 1.000000000000000000, -0.000000000000000000 ) ) ;
#14083=CARTESIAN_POINT ( 'NONE',  ( 30.42502041961813575, 271.1055109169419097, 20.00000000000000355 ) ) ;
#14088=AXIS2_PLACEMENT_3D ( 'NONE', #18650, #15331, #10321 ) ;
#14089=VERTEX_POINT ( 'NONE', #8716 ) ;
#14091=ORIENTED_EDGE ( 'NONE', *, *, #199, .T. ) ;
#14093=DIRECTION ( 'NONE',  ( -9.855701800883827197E-17, 1.000000000000000000, 9.855701800883827197E-17 ) ) ;
#14098=CARTESIAN_POINT ( 'NONE',  ( 125.7989814974898337, 160.1716627696691830, -40.00000000000000000 ) ) ;
#14125=ADVANCED_FACE ( 'NONE', ( #20616 ), #8823, .F. ) ;
#14128=CARTESIAN_POINT ( 'NONE',  ( 20.42502041961806825, 281.1055109169419666, -20.00000000000000355 ) ) ;
#14131=ADVANCED_FACE ( 'NONE', ( #18660 ), #19103, .T. ) ;
#14133=LINE ( 'NONE', #10968, #2660 ) ;
#14136=AXIS2_PLACEMENT_3D ( 'NONE', #19483, #12783, #16249 ) ;
#14144=CARTESIAN_POINT ( 'NONE',  ( 51.50493485826542184, 170.1716627696692683, -20.00000000000000355 ) ) ;
#14155=DIRECTION ( 'NONE',  ( 0.000000000000000000, -0.000000000000000000, 1.000000000000000000 ) ) ;
#14158=CARTESIAN_POINT ( 'NONE',  ( 91.21585410611801592, 31.85652257517428865, 85.46735025547120301 ) ) ;
#14161=AXIS2_PLACEMENT_3D ( 'NONE', #12947, #6433, #9478 ) ;
#14164=DIRECTION ( 'NONE',  ( 0.000000000000000000, 0.000000000000000000, -1.000000000000000000 ) ) ;
#14165=CARTESIAN_POINT ( 'NONE',  ( 78.68120802659203150, 149.7457237375499517, -40.00000000000000000 ) ) ;
#14170=ORIENTED_EDGE ( 'NONE', *, *, #9485, .F. ) ;
#14171=DIRECTION ( 'NONE',  ( 0.9283449136418786551, 0.000000000000000000, 0.3717199501173604759 ) ) ;
#14172=ORIENTED_EDGE ( 'NONE', *, *, #8688, .F. ) ;
#14173=ORIENTED_EDGE ( 'NONE', *, *, #9452, .T. ) ;
#14183=LINE ( 'NONE', #8969, #15201 ) ;
#14192=ORIENTED_EDGE ( 'NONE', *, *, #14654, .F. ) ;
#14197=VERTEX_POINT ( 'NONE', #19520 ) ;
#14203=DIRECTION ( 'NONE',  ( 0.000000000000000000, 0.000000000000000000, -1.000000000000000000 ) ) ;
#14204=VECTOR ( 'NONE', #998, 1000.000000000000000 ) ;
#14210=EDGE_CURVE ( 'NONE', #18850, #14441, #6007, .T. ) ;
#14215=DIRECTION ( 'NONE',  ( 0.000000000000000000, 0.000000000000000000, -1.000000000000000000 ) ) ;
#14218=AXIS2_PLACEMENT_3D ( 'NONE', #20153, #5321, #19831 ) ;
#14224=ADVANCED_FACE ( 'NONE', ( #4599, #17892 ), #14675, .F. ) ;
#14225=ORIENTED_EDGE ( 'NONE', *, *, #7618, .F. ) ;
#14231=DIRECTION ( 'NONE',  ( 0.000000000000000000, 1.000000000000000000, 0.000000000000000000 ) ) ;
#14239=STYLED_ITEM('',(#21414),#11152);
#14245=DIRECTION ( 'NONE',  ( -0.000000000000000000, -0.000000000000000000, 1.000000000000000000 ) ) ;
#14248=FACE_OUTER_BOUND ( 'NONE', #680, .T. ) ;
#14252=ORIENTED_EDGE ( 'NONE', *, *, #8610, .T. ) ;
#14255=VERTEX_POINT ( 'NONE', #2775 ) ;
#14258=ORIENTED_EDGE ( 'NONE', *, *, #2446, .F. ) ;
#14265=DIRECTION ( 'NONE',  ( 0.000000000000000000, -0.000000000000000000, 1.000000000000000000 ) ) ;
#14269=FACE_OUTER_BOUND ( 'NONE', #7141, .T. ) ;
#14271=EDGE_CURVE ( 'NONE', #4211, #2296, #2984, .T. ) ;
#14277=DIRECTION ( 'NONE',  ( -0.000000000000000000, -0.000000000000000000, 1.000000000000000000 ) ) ;
#14291=ORIENTED_EDGE ( 'NONE', *, *, #10354, .T. ) ;
#14304=ORIENTED_EDGE ( 'NONE', *, *, #15892, .F. ) ;
#14307=ORIENTED_EDGE ( 'NONE', *, *, #1982, .T. ) ;
#14309=ORIENTED_EDGE ( 'NONE', *, *, #20004, .F. ) ;
#14329=VECTOR ( 'NONE', #14866, 1000.000000000000000 ) ;
#14332=( BOUNDED_CURVE ( )  B_SPLINE_CURVE ( 3, ( #13944, #2362, #15565, #4191 ),
 .UNSPECIFIED., .F., .T. ) 
 B_SPLINE_CURVE_WITH_KNOTS ( ( 4, 4 ),
 ( 3.164427803482926738, 4.453488305187281782 ),
 .UNSPECIFIED. ) 
 CURVE ( )  GEOMETRIC_REPRESENTATION_ITEM ( )  RATIONAL_B_SPLINE_CURVE ( ( 1.000000000000000000, 0.8662547274802335773, 0.8662547274802335773, 1.000000000000000000 ) ) 
 REPRESENTATION_ITEM ( '' )  );
#14335=EDGE_CURVE ( 'NONE', #14726, #16087, #19845, .T. ) ;
#14338=ORIENTED_EDGE ( 'NONE', *, *, #2940, .F. ) ;
#14352=EDGE_CURVE ( 'NONE', #10230, #18299, #13471, .T. ) ;
#14353=CARTESIAN_POINT ( 'NONE',  ( 52.60622592008805043, 30.52886280891152282, -151.0302712373927250 ) ) ;
#14354=CARTESIAN_POINT ( 'NONE',  ( 20.42502041961806825, 281.1055109169419666, 20.00000000000000355 ) ) ;
#14375=DIRECTION ( 'NONE',  ( -0.000000000000000000, -0.000000000000000000, 1.000000000000000000 ) ) ;
#14382=CARTESIAN_POINT ( 'NONE',  ( 51.98438129372387806, 56.85652257517428865, -94.99999999999994316 ) ) ;
#14390=ORIENTED_EDGE ( 'NONE', *, *, #1749, .T. ) ;
#14392=DIRECTION ( 'NONE',  ( -0.000000000000000000, -0.000000000000000000, -1.000000000000000000 ) ) ;
#14399=CYLINDRICAL_SURFACE ( 'NONE', #2408, 9.999999999999994671 ) ;
#14401=EDGE_CURVE ( 'NONE', #9753, #19163, #19734, .T. ) ;
#14404=AXIS2_PLACEMENT_3D ( 'NONE', #2209, #18528, #5655 ) ;
#14408=AXIS2_PLACEMENT_3D ( 'NONE', #1877, #8446, #4388 ) ;
#14410=DIRECTION ( 'NONE',  ( 1.000000000000000000, 0.000000000000000000, 0.000000000000000000 ) ) ;
#14415=ORIENTED_EDGE ( 'NONE', *, *, #7363, .F. ) ;
#14424=FACE_OUTER_BOUND ( 'NONE', #8637, .T. ) ;
#14426=AXIS2_PLACEMENT_3D ( 'NONE', #1152, #15862, #9560 ) ;
#14441=VERTEX_POINT ( 'NONE', #70 ) ;
#14449=CARTESIAN_POINT ( 'NONE',  ( -18.68588794268873698, 281.1055109169419666, -40.00000000000000000 ) ) ;
#14455=ADVANCED_FACE ( 'NONE', ( #3511 ), #13258, .F. ) ;
#14468=EDGE_CURVE ( 'NONE', #6673, #3284, #19106, .T. ) ;
#14469=ORIENTED_EDGE ( 'NONE', *, *, #9152, .F. ) ;
#14472=VERTEX_POINT ( 'NONE', #18742 ) ;
#14474=CYLINDRICAL_SURFACE ( 'NONE', #7903, 40.00000000000000000 ) ;
#14478=LINE ( 'NONE', #4935, #8022 ) ;
#14480=AXIS2_PLACEMENT_3D ( 'NONE', #4820, #7949, #11416 ) ;
#14482=CARTESIAN_POINT ( 'NONE',  ( -49.57497958038185715, 160.1716627696692683, -60.00000000000000000 ) ) ;
#14486=DIRECTION ( 'NONE',  ( 1.000000000000000000, 0.000000000000000000, 0.000000000000000000 ) ) ;
#14495=CARTESIAN_POINT ( 'NONE',  ( 79.78925230247502043, 142.5259582928263455, 20.00000000000000355 ) ) ;
#14509=DIRECTION ( 'NONE',  ( 0.000000000000000000, 1.000000000000000000, 0.000000000000000000 ) ) ;
#14510=ORIENTED_EDGE ( 'NONE', *, *, #19182, .F. ) ;
#14513=ORIENTED_EDGE ( 'NONE', *, *, #6988, .T. ) ;
#14514=ORIENTED_EDGE ( 'NONE', *, *, #18995, .F. ) ;
#14525=DIRECTION ( 'NONE',  ( -0.000000000000000000, -0.000000000000000000, -1.000000000000000000 ) ) ;
#14532=LINE ( 'NONE', #15837, #11269 ) ;
#14538=AXIS2_PLACEMENT_3D ( 'NONE', #14018, #20597, #17357 ) ;
#14541=CIRCLE ( 'NONE', #7933, 10.00000000000000533 ) ;
#14546=ORIENTED_EDGE ( 'NONE', *, *, #1355, .T. ) ;
#14549=CARTESIAN_POINT ( 'NONE',  ( 115.7989814974898337, 142.5259582928263455, -20.00000000000000355 ) ) ;
#14552=CARTESIAN_POINT ( 'NONE',  ( -15.91779735428318787, 47.19211360595399896, 47.93839540604061256 ) ) ;
#14553=DIRECTION ( 'NONE',  ( 0.000000000000000000, 1.000000000000000000, 0.000000000000000000 ) ) ;
#14554=DIRECTION ( 'NONE',  ( -9.855701800883827197E-17, 1.000000000000000000, 0.000000000000000000 ) ) ;
#14555=DIRECTION ( 'NONE',  ( -1.000000000000000000, 0.000000000000000000, 0.000000000000000000 ) ) ;
#14557=CIRCLE ( 'NONE', #10039, 4.000000000000003553 ) ;
#14558=FACE_OUTER_BOUND ( 'NONE', #961, .T. ) ;
#14559=VECTOR ( 'NONE', #21226, 1000.000000000000000 ) ;
#14565=ORIENTED_EDGE ( 'NONE', *, *, #9538, .T. ) ;
#14567=DIRECTION ( 'NONE',  ( 0.1337298367054296222, -0.9910178256594273094, 0.000000000000000000 ) ) ;
#14572=VECTOR ( 'NONE', #14392, 1000.000000000000000 ) ;
#14577=FACE_OUTER_BOUND ( 'NONE', #8149, .T. ) ;
#14579=CARTESIAN_POINT ( 'NONE',  ( 78.68120802659203150, 149.7457237375499517, 94.99999999999994316 ) ) ;
#14580=EDGE_CURVE ( 'NONE', #18698, #1447, #596, .T. ) ;
#14584=CYLINDRICAL_SURFACE ( 'NONE', #16393, 4.000000000000001776 ) ;
#14587=FACE_OUTER_BOUND ( 'NONE', #3727, .T. ) ;
#14592=VECTOR ( 'NONE', #12202, 1000.000000000000000 ) ;
#14599=ORIENTED_EDGE ( 'NONE', *, *, #2295, .T. ) ;
#14602=ORIENTED_EDGE ( 'NONE', *, *, #3210, .T. ) ;
#14609=CARTESIAN_POINT ( 'NONE',  ( 81.24038404635966515, -343.0245277843623057, 94.99999999999994316 ) ) ;
#14617=DIRECTION ( 'NONE',  ( -0.9283449136418786551, -0.000000000000000000, -0.3717199501173604204 ) ) ;
#14624=EDGE_LOOP ( 'NONE', ( #7457, #5000, #17639, #3466, #19296 ) ) ;
#14628=CARTESIAN_POINT ( 'NONE',  ( -28.68588794268874054, 333.8848358243226357, -40.00000000000000000 ) ) ;
#14633=VECTOR ( 'NONE', #18606, 1000.000000000000000 ) ;
#14641=CARTESIAN_POINT ( 'NONE',  ( 35.96497763894179656, 163.7662197624121916, 60.00000000000000000 ) ) ;
#14646=AXIS2_PLACEMENT_3D ( 'NONE', #2548, #1150, #834 ) ;
#14650=FACE_OUTER_BOUND ( 'NONE', #3089, .T. ) ;
#14651=ORIENTED_EDGE ( 'NONE', *, *, #3555, .F. ) ;
#14652=DIRECTION ( 'NONE',  ( 0.000000000000000000, 1.000000000000000000, 0.000000000000000000 ) ) ;
#14653=ADVANCED_FACE ( 'NONE', ( #20588 ), #7273, .T. ) ;
#14654=EDGE_CURVE ( 'NONE', #1580, #18169, #6099, .T. ) ;
#14657=DIRECTION ( 'NONE',  ( -0.000000000000000000, -0.000000000000000000, -1.000000000000000000 ) ) ;
#14661=CARTESIAN_POINT ( 'NONE',  ( -28.68588794268873698, -129.7637193493918915, 49.60091809715359545 ) ) ;
#14666=FACE_OUTER_BOUND ( 'NONE', #1137, .T. ) ;
#14667=CIRCLE ( 'NONE', #18447, 40.00000000000000000 ) ;
#14669=EDGE_CURVE ( 'NONE', #7864, #17482, #11937, .T. ) ;
#14670=CARTESIAN_POINT ( 'NONE',  ( 20.42502041961813930, 230.5765313837437418, 40.00000000000000000 ) ) ;
#14671=LINE ( 'NONE', #2770, #4180 ) ;
#14675=PLANE ( 'NONE',  #3682 ) ;
#14686=ORIENTED_EDGE ( 'NONE', *, *, #13291, .F. ) ;
#14691=DIRECTION ( 'NONE',  ( -0.000000000000000000, -0.000000000000000000, -1.000000000000000000 ) ) ;
#14693=CARTESIAN_POINT ( 'NONE',  ( 72.94945500224395118, 285.0140030772282103, -20.00000000000000355 ) ) ;
#14699=CYLINDRICAL_SURFACE ( 'NONE', #18885, 125.0000000000000000 ) ;
#14709=ORIENTED_EDGE ( 'NONE', *, *, #10926, .T. ) ;
#14714=CARTESIAN_POINT ( 'NONE',  ( 72.94945500224395118, 285.0140030772282103, 40.00000000000000000 ) ) ;
#14715=DIRECTION ( 'NONE',  ( 0.000000000000000000, -1.000000000000000000, 0.000000000000000000 ) ) ;
#14722=FACE_OUTER_BOUND ( 'NONE', #8719, .T. ) ;
#14723=ORIENTED_EDGE ( 'NONE', *, *, #14335, .F. ) ;
#14726=VERTEX_POINT ( 'NONE', #18125 ) ;
#14727=CARTESIAN_POINT ( 'NONE',  ( 0.000000000000000000, 0.000000000000000000, -60.00000000000000000 ) ) ;
#14730=EDGE_CURVE ( 'NONE', #4363, #2506, #17863, .T. ) ;
#14743=EDGE_CURVE ( 'NONE', #1580, #10233, #3213, .T. ) ;
#14745=CARTESIAN_POINT ( 'NONE',  ( -33.54679760364381025, 54.20929210266576348, 120.4143613387277867 ) ) ;
#14751=VERTEX_POINT ( 'NONE', #5150 ) ;
#14756=CARTESIAN_POINT ( 'NONE',  ( -162.2727221670389781, 10.52886280891152104, -4.999999999999990230 ) ) ;
#14758=DIRECTION ( 'NONE',  ( 0.000000000000000000, 0.000000000000000000, 1.000000000000000000 ) ) ;
#14765=CARTESIAN_POINT ( 'NONE',  ( -24.59534672197139216, 45.54211327328065551, 49.43263578720818430 ) ) ;
#14767=CARTESIAN_POINT ( 'NONE',  ( -18.68588794268873698, 281.1055109169419666, 20.00000000000000355 ) ) ;
#14770=CARTESIAN_POINT ( 'NONE',  ( -28.68588794268873343, 47.23886018424757083, 49.60091809715359545 ) ) ;
#14775=DIRECTION ( 'NONE',  ( -0.9999562017632421806, 0.000000000000000000, -0.009359196291876339252 ) ) ;
#14783=CIRCLE ( 'NONE', #21331, 43.46661168214937732 ) ;
#14784=ORIENTED_EDGE ( 'NONE', *, *, #7105, .T. ) ;
#14790=EDGE_CURVE ( 'NONE', #5025, #8699, #18019, .T. ) ;
#14793=CIRCLE ( 'NONE', #21338, 4.999999999999990230 ) ;
#14795=LINE ( 'NONE', #14579, #19644 ) ;
#14796=CARTESIAN_POINT ( 'NONE',  ( 79.78925230247502043, 142.5259582928263455, 40.00000000000000000 ) ) ;
#14799=FACE_OUTER_BOUND ( 'NONE', #17744, .T. ) ;
#14803=ADVANCED_FACE ( 'NONE', ( #3529 ), #16739, .F. ) ;
#14810=DIRECTION ( 'NONE',  ( -1.000000000000000000, 0.000000000000000000, 0.000000000000000000 ) ) ;
#14811=ORIENTED_EDGE ( 'NONE', *, *, #2364, .F. ) ;
#14815=ORIENTED_EDGE ( 'NONE', *, *, #18779, .T. ) ;
#14824=CARTESIAN_POINT ( 'NONE',  ( 28.16023193154655502, 323.8848358243226357, -20.00000000000000355 ) ) ;
#14826=LINE ( 'NONE', #9720, #20847 ) ;
#14827=VECTOR ( 'NONE', #18760, 1000.000000000000000 ) ;
#14829=UNCERTAINTY_MEASURE_WITH_UNIT (LENGTH_MEASURE( 1.000000000000000082E-05 ), #16111, 'distance_accuracy_value', 'NONE');
#14836=ORIENTED_EDGE ( 'NONE', *, *, #15056, .T. ) ;
#14839=CARTESIAN_POINT ( 'NONE',  ( -49.57497958038186425, 230.5765313837437418, -60.00000000000000000 ) ) ;
#14863=ORIENTED_EDGE ( 'NONE', *, *, #5247, .F. ) ;
#14864=PLANE ( 'NONE',  #1508 ) ;
#14865=ORIENTED_EDGE ( 'NONE', *, *, #16102, .T. ) ;
#14866=DIRECTION ( 'NONE',  ( -0.000000000000000000, -0.000000000000000000, 1.000000000000000000 ) ) ;
#14867=EDGE_CURVE ( 'NONE', #9937, #3730, #1296, .T. ) ;
#14873=CARTESIAN_POINT ( 'NONE',  ( 29.72350413846044859, 280.4463447002762564, 20.00000000000000355 ) ) ;
#14875=CARTESIAN_POINT ( 'NONE',  ( -10.94825334483056345, 54.75396031329337632, 46.32098196382629141 ) ) ;
#14883=EDGE_CURVE ( 'NONE', #7551, #1161, #12061, .T. ) ;
#14889=ORIENTED_EDGE ( 'NONE', *, *, #9276, .T. ) ;
#14892=ADVANCED_FACE ( 'NONE', ( #8596 ), #5353, .F. ) ;
#14894=CARTESIAN_POINT ( 'NONE',  ( 91.21585410611801592, 56.85652257517427444, 40.00000000000000000 ) ) ;
#14902=VECTOR ( 'NONE', #1874, 1000.000000000000000 ) ;
#14907=CARTESIAN_POINT ( 'NONE',  ( 125.7989814974898053, 10.52886280891152104, -40.00000000000000000 ) ) ;
#14912=DIRECTION ( 'NONE',  ( 0.000000000000000000, 0.000000000000000000, -1.000000000000000000 ) ) ;
#14921=EDGE_CURVE ( 'NONE', #10498, #19453, #16945, .T. ) ;
#14927=CARTESIAN_POINT ( 'NONE',  ( 82.89408817951444064, 286.0648460576640559, 40.00000000000000000 ) ) ;
#14928=CARTESIAN_POINT ( 'NONE',  ( 118.4271928232701043, 31.85652257517428865, -40.00000000000000000 ) ) ;
#14929=AXIS2_PLACEMENT_3D ( 'NONE', #14495, #4735, #7971 ) ;
#14933=DIRECTION ( 'NONE',  ( 1.232945044042657126E-32, -9.855701800883825964E-17, 1.000000000000000000 ) ) ;
#14944=CARTESIAN_POINT ( 'NONE',  ( -18.68588794268873698, 323.8848358243226357, -20.00000000000000355 ) ) ;
#14946=VERTEX_POINT ( 'NONE', #8813 ) ;
#14954=AXIS2_PLACEMENT_3D ( 'NONE', #20930, #21034, #19200 ) ;
#14960=LINE ( 'NONE', #4994, #15781 ) ;
#14968=VERTEX_POINT ( 'NONE', #20185 ) ;
#14981=DIRECTION ( 'NONE',  ( 0.000000000000000000, -1.000000000000000000, 0.000000000000000000 ) ) ;
#14982=DIRECTION ( 'NONE',  ( -0.9910178256594274204, -0.1337298367054296500, 0.000000000000000000 ) ) ;
#14987=DIRECTION ( 'NONE',  ( 0.000000000000000000, -0.000000000000000000, 1.000000000000000000 ) ) ;
#14996=ORIENTED_EDGE ( 'NONE', *, *, #5260, .F. ) ;
#14998=ORIENTED_EDGE ( 'NONE', *, *, #11658, .F. ) ;
#15002=ORIENTED_EDGE ( 'NONE', *, *, #4123, .T. ) ;
#15007=CARTESIAN_POINT ( 'NONE',  ( -12.55404211795046798, 50.68295084878040058, -46.90452445606911880 ) ) ;
#15008=VECTOR ( 'NONE', #19643, 1000.000000000000000 ) ;
#15012=CARTESIAN_POINT ( 'NONE',  ( 81.24038404635966515, 30.52886280891152282, 94.99999999999994316 ) ) ;
#15015=CARTESIAN_POINT ( 'NONE',  ( -33.73083959248491226, 54.96237515877132296, 49.34423148476142984 ) ) ;
#15023=AXIS2_PLACEMENT_3D ( 'NONE', #16271, #14652, #14758 ) ;
#15027=DIRECTION ( 'NONE',  ( 1.000000000000000000, 0.000000000000000000, 0.000000000000000000 ) ) ;
#15028=ORIENTED_EDGE ( 'NONE', *, *, #3138, .T. ) ;
#15032=VERTEX_POINT ( 'NONE', #3949 ) ;
#15044=EDGE_CURVE ( 'NONE', #5103, #3984, #10642, .T. ) ;
#15047=VERTEX_POINT ( 'NONE', #10534 ) ;
#15049=ORIENTED_EDGE ( 'NONE', *, *, #607, .T. ) ;
#15050=VECTOR ( 'NONE', #10465, 1000.000000000000000 ) ;
#15056=EDGE_CURVE ( 'NONE', #8313, #16730, #8876, .T. ) ;
#15063=DIRECTION ( 'NONE',  ( 1.000000000000000000, 0.000000000000000000, 0.000000000000000000 ) ) ;
#15065=DIRECTION ( 'NONE',  ( 0.000000000000000000, 0.000000000000000000, 1.000000000000000000 ) ) ;
#15069=CARTESIAN_POINT ( 'NONE',  ( 71.15180554307954708, 205.5430855047783041, -43.20892846146212918 ) ) ;
#15071=EDGE_CURVE ( 'NONE', #10361, #10687, #17366, .T. ) ;
#15074=ORIENTED_EDGE ( 'NONE', *, *, #8077, .F. ) ;
#15077=VERTEX_POINT ( 'NONE', #14128 ) ;
#15079=ORIENTED_EDGE ( 'NONE', *, *, #2280, .F. ) ;
#15090=LINE ( 'NONE', #6949, #9971 ) ;
#15102=VECTOR ( 'NONE', #2345, 1000.000000000000000 ) ;
#15103=VERTEX_POINT ( 'NONE', #9129 ) ;
#15108=DIRECTION ( 'NONE',  ( 1.000000000000000000, 0.000000000000000000, 0.000000000000000000 ) ) ;
#15111=ORIENTED_EDGE ( 'NONE', *, *, #18476, .T. ) ;
#15113=CARTESIAN_POINT ( 'NONE',  ( -10.76731745429010090, 56.85652257517428865, -46.25122601329427141 ) ) ;
#15117=DIRECTION ( 'NONE',  ( 0.000000000000000000, 0.000000000000000000, 1.000000000000000000 ) ) ;
#15123=LINE ( 'NONE', #5356, #19411 ) ;
#15128=FACE_OUTER_BOUND ( 'NONE', #11661, .T. ) ;
#15130=ADVANCED_FACE ( 'NONE', ( #4589 ), #20928, .T. ) ;
#15133=DIRECTION ( 'NONE',  ( 0.000000000000000000, 0.000000000000000000, -1.000000000000000000 ) ) ;
#15140=EDGE_LOOP ( 'NONE', ( #10256, #13373, #9171, #7169 ) ) ;
#15142=EDGE_CURVE ( 'NONE', #454, #17590, #4377, .T. ) ;
#15169=VECTOR ( 'NONE', #4512, 1000.000000000000000 ) ;
#15170=CARTESIAN_POINT ( 'NONE',  ( -23.06654969220458895, 45.31613216062292082, 122.8557246090902026 ) ) ;
#15171=LINE ( 'NONE', #13113, #20081 ) ;
#15182=CARTESIAN_POINT ( 'NONE',  ( 20.42502041961813575, 271.1055109169419666, 40.00000000000000000 ) ) ;
#15184=AXIS2_PLACEMENT_3D ( 'NONE', #8998, #806, #20902 ) ;
#15194=DIRECTION ( 'NONE',  ( 0.000000000000000000, -1.000000000000000000, 0.000000000000000000 ) ) ;
#15201=VECTOR ( 'NONE', #779, 1000.000000000000000 ) ;
#15203=DIRECTION ( 'NONE',  ( -1.000000000000000000, -0.000000000000000000, -0.000000000000000000 ) ) ;
#15209=EDGE_LOOP ( 'NONE', ( #3038, #4236, #20591, #7279, #2666, #11351 ) ) ;
#15211=EDGE_LOOP ( 'NONE', ( #10391, #21334, #15452, #10474, #20787, #16650, #9116 ) ) ;
#15216=DIRECTION ( 'NONE',  ( 0.000000000000000000, 0.000000000000000000, -1.000000000000000000 ) ) ;
#15218=LINE ( 'NONE', #18649, #3411 ) ;
#15222=PLANE ( 'NONE',  #10071 ) ;
#15229=ORIENTED_EDGE ( 'NONE', *, *, #4546, .F. ) ;
#15235=ORIENTED_EDGE ( 'NONE', *, *, #8471, .F. ) ;
#15237=EDGE_CURVE ( 'NONE', #5798, #12056, #18209, .T. ) ;
#15238=LINE ( 'NONE', #428, #17629 ) ;
#15240=AXIS2_PLACEMENT_3D ( 'NONE', #19373, #8297, #4559 ) ;
#15241=ORIENTED_EDGE ( 'NONE', *, *, #1256, .T. ) ;
#15244=FACE_OUTER_BOUND ( 'NONE', #16010, .T. ) ;
#15247=CARTESIAN_POINT ( 'NONE',  ( 51.50493485826542894, 160.1716627696692683, 61.61851857202071869 ) ) ;
#15252=AXIS2_PLACEMENT_3D ( 'NONE', #13017, #14657, #4479 ) ;
#15255=B_SPLINE_CURVE_WITH_KNOTS ( 'NONE', 3,
 ( #3270, #1541, #8112, #14745, #4882, #9845, #28, #13435, #1873, #11799, #18396, #10485, #6922, #3583, #11905, #10063, #7237, #7029, #464, #2181, #20027, #13651, #15170, #20236 ),
 .UNSPECIFIED., .F., .F.,
 ( 4, 2, 2, 2, 2, 2, 2, 2, 2, 2, 2, 4 ),
 ( 2.860979249076398407E-17, 0.002281674285428699801, 0.003422511428143036692, 0.004563348570857373582, 0.006845022856286023076, 0.007985859999000345655, 0.009126697141714665631, 0.01140837142714332640, 0.01369004571257198544, 0.01483088285528631235, 0.01597171999800063927, 0.01825339428342929657 ),
 .UNSPECIFIED. ) ;
#15263=ORIENTED_EDGE ( 'NONE', *, *, #4201, .F. ) ;
#15270=ORIENTED_EDGE ( 'NONE', *, *, #3235, .T. ) ;
#15282=CARTESIAN_POINT ( 'NONE',  ( 6.416697501590670427, 217.7548513357008630, 49.99999999999999289 ) ) ;
#15283=ADVANCED_FACE ( 'NONE', ( #19512, #17678, #13135 ), #13355, .F. ) ;
#15291=CARTESIAN_POINT ( 'NONE',  ( 75.04415151326509203, 162.3117964647028373, -60.96179693900064933 ) ) ;
#15302=CYLINDRICAL_SURFACE ( 'NONE', #12409, 11.54039041455135184 ) ;
#15304=VECTOR ( 'NONE', #970, 1000.000000000000000 ) ;
#15307=CARTESIAN_POINT ( 'NONE',  ( 29.72350413846044859, 280.4463447002762564, -20.00000000000000355 ) ) ;
#15311=CARTESIAN_POINT ( 'NONE',  ( -29.29923972067796356, 47.64464476306663698, -121.5194033971115601 ) ) ;
#15316=ADVANCED_FACE ( 'NONE', ( #1899 ), #4907, .F. ) ;
#15324=VERTEX_POINT ( 'NONE', #59 ) ;
#15326=CARTESIAN_POINT ( 'NONE',  ( -15.94757079417145462, 47.22349452202089282, -47.93784354121613234 ) ) ;
#15330=CARTESIAN_POINT ( 'NONE',  ( 125.7989814974898337, 160.1716627696691830, 40.00000000000000000 ) ) ;
#15331=DIRECTION ( 'NONE',  ( 0.000000000000000000, -1.000000000000000000, 0.000000000000000000 ) ) ;
#15333=CARTESIAN_POINT ( 'NONE',  ( 91.21585410611801592, 56.85652257517428865, 94.99999999999994316 ) ) ;
#15334=VECTOR ( 'NONE', #8657, 1000.000000000000000 ) ;
#15337=CARTESIAN_POINT ( 'NONE',  ( 2.416697501590669095, 217.7548513357008630, 60.00000000000000000 ) ) ;
#15344=AXIS2_PLACEMENT_3D ( 'NONE', #20918, #12375, #4147 ) ;
#15345=ORIENTED_EDGE ( 'NONE', *, *, #14790, .F. ) ;
#15363=CARTESIAN_POINT ( 'NONE',  ( -49.57497958038185715, 160.1716627696692683, -50.00000000000000000 ) ) ;
#15364=ADVANCED_FACE ( 'NONE', ( #9869 ), #6844, .F. ) ;
#15368=ORIENTED_EDGE ( 'NONE', *, *, #12350, .T. ) ;
#15370=ORIENTED_EDGE ( 'NONE', *, *, #3816, .T. ) ;
#15371=EDGE_LOOP ( 'NONE', ( #5075, #5823, #18889, #20670 ) ) ;
#15381=CARTESIAN_POINT ( 'NONE',  ( -162.2727221670389781, 30.52886280891152282, -20.57735571454641033 ) ) ;
#15385=CARTESIAN_POINT ( 'NONE',  ( 28.16023193154655502, 323.8848358243226357, 40.00000000000000000 ) ) ;
#15389=ORIENTED_EDGE ( 'NONE', *, *, #6426, .F. ) ;
#15395=CARTESIAN_POINT ( 'NONE',  ( 78.68120802659203150, 149.7457237375499517, -66.14548919766382085 ) ) ;
#15398=DIRECTION ( 'NONE',  ( 0.02283316540262222277, -0.9997392892938120612, -0.000000000000000000 ) ) ;
#15411=CARTESIAN_POINT ( 'NONE',  ( 81.24038404635966515, 30.52886280891152282, 94.99999999999994316 ) ) ;
#15412=DIRECTION ( 'NONE',  ( -0.4989387216749512355, -0.8666372666885295839, -0.000000000000000000 ) ) ;
#15414=DIRECTION ( 'NONE',  ( 3.836511174089486173E-16, -0.000000000000000000, 1.000000000000000000 ) ) ;
#15420=CARTESIAN_POINT ( 'NONE',  ( 51.50493485826542184, 170.1716627696692683, 57.52045949366692668 ) ) ;
#15422=DIRECTION ( 'NONE',  ( -0.000000000000000000, -0.000000000000000000, -1.000000000000000000 ) ) ;
#15425=ORIENTED_EDGE ( 'NONE', *, *, #10583, .T. ) ;
#15427=CARTESIAN_POINT ( 'NONE',  ( 60.03793209889851568, 10.52886280891152104, -152.3753892284480003 ) ) ;
#15435=DIRECTION ( 'NONE',  ( -8.901024030850960568E-17, 0.000000000000000000, 1.000000000000000000 ) ) ;
#15440=CARTESIAN_POINT ( 'NONE',  ( 30.42502041961814996, 170.1716627696692683, 20.00000000000000355 ) ) ;
#15442=EDGE_CURVE ( 'NONE', #17480, #11300, #13395, .T. ) ;
#15443=EDGE_LOOP ( 'NONE', ( #19240, #17532, #20653, #17144 ) ) ;
#15447=EDGE_CURVE ( 'NONE', #18701, #19677, #9717, .T. ) ;
#15448=AXIS2_PLACEMENT_3D ( 'NONE', #12263, #10412, #7061 ) ;
#15452=ORIENTED_EDGE ( 'NONE', *, *, #14669, .F. ) ;
#15453=AXIS2_PLACEMENT_3D ( 'NONE', #16607, #8364, #14987 ) ;
#15458=EDGE_CURVE ( 'NONE', #5025, #11304, #7981, .T. ) ;
#15464=CARTESIAN_POINT ( 'NONE',  ( 91.21585410611801592, 31.85652257517428865, -85.46735025547123143 ) ) ;
#15467=LINE ( 'NONE', #2371, #13274 ) ;
#15469=ORIENTED_EDGE ( 'NONE', *, *, #18476, .F. ) ;
#15484=DIRECTION ( 'NONE',  ( 0.000000000000000000, 0.000000000000000000, 1.000000000000000000 ) ) ;
#15494=EDGE_CURVE ( 'NONE', #13185, #7305, #4847, .T. ) ;
#15497=VERTEX_POINT ( 'NONE', #13082 ) ;
#15511=DIRECTION ( 'NONE',  ( 1.000000000000000000, 0.000000000000000000, 0.000000000000000000 ) ) ;
#15533=ORIENTED_EDGE ( 'NONE', *, *, #17728, .F. ) ;
#15537=DIRECTION ( 'NONE',  ( 0.000000000000000000, -1.000000000000000000, 0.000000000000000000 ) ) ;
#15538=DIRECTION ( 'NONE',  ( 0.000000000000000000, 0.000000000000000000, 1.000000000000000000 ) ) ;
#15541=FACE_OUTER_BOUND ( 'NONE', #1032, .T. ) ;
#15544=CARTESIAN_POINT ( 'NONE',  ( 20.42502041961813930, 230.5765313837437418, -40.00000000000000000 ) ) ;
#15554=ORIENTED_EDGE ( 'NONE', *, *, #16571, .F. ) ;
#15558=ORIENTED_EDGE ( 'NONE', *, *, #15142, .F. ) ;
#15561=VERTEX_POINT ( 'NONE', #6150 ) ;
#15562=DIRECTION ( 'NONE',  ( 1.000000000000000000, 0.000000000000000000, 0.000000000000000000 ) ) ;
#15565=CARTESIAN_POINT ( 'NONE',  ( 75.04415151326509203, 162.3117964647028373, 60.96179693900064933 ) ) ;
#15566=DIRECTION ( 'NONE',  ( -1.250996701150283068E-16, 1.000000000000000000, 0.000000000000000000 ) ) ;
#15568=DIRECTION ( 'NONE',  ( -0.000000000000000000, 1.000000000000000000, -0.000000000000000000 ) ) ;
#15578=EDGE_CURVE ( 'NONE', #6060, #19853, #14783, .T. ) ;
#15579=ORIENTED_EDGE ( 'NONE', *, *, #4761, .F. ) ;
#15580=DIRECTION ( 'NONE',  ( -0.000000000000000000, -0.000000000000000000, 1.000000000000000000 ) ) ;
#15584=DIRECTION ( 'NONE',  ( 1.000000000000000000, 0.000000000000000000, 0.000000000000000000 ) ) ;
#15588=PRODUCT_DEFINITION_FORMATION_WITH_SPECIFIED_SOURCE ( 'ANY', '', #4407, .NOT_KNOWN. ) ;
#15594=AXIS2_PLACEMENT_3D ( 'NONE', #4462, #17551, #12902 ) ;
#15598=LINE ( 'NONE', #4435, #10608 ) ;
#15599=CARTESIAN_POINT ( 'NONE',  ( 52.60622592008805043, 30.52886280891152282, -151.0302712373927250 ) ) ;
#15603=VERTEX_POINT ( 'NONE', #15544 ) ;
#15606=ORIENTED_EDGE ( 'NONE', *, *, #1234, .F. ) ;
#15607=VERTEX_POINT ( 'NONE', #13919 ) ;
#15622=DIRECTION ( 'NONE',  ( -0.000000000000000000, -0.000000000000000000, -1.000000000000000000 ) ) ;
#15624=VECTOR ( 'NONE', #8183, 1000.000000000000000 ) ;
#15629=B_SPLINE_CURVE_WITH_KNOTS ( 'NONE', 3,
 ( #1457, #16282, #12922, #3399, #19511, #1564, #11502, #2976, #8246, #19723, #14765, #21138, #4690, #11612, #11182, #9764, #11284, #21244, #5012, #8134, #16493, #14552, #6738, #6409, #13023, #9980, #19615, #21351, #1675, #9554, #14875, #19836, #18203, #4792 ),
 .UNSPECIFIED., .F., .F.,
 ( 4, 2, 2, 2, 2, 2, 2, 2, 2, 2, 2, 2, 2, 2, 2, 2, 4 ),
 ( 0.01132186211905188838, 0.01210437382053968641, 0.01288688552202748618, 0.01445190892500309264, 0.01523442062649089240, 0.01601693232797869390, 0.01758195573095429343, 0.01914697913392988948, 0.02071200253690548554, 0.02227702593988108160, 0.02384204934285668112, 0.02697209614880787670, 0.03010214295475907922, 0.03166716635773467875, 0.03323218976071028175, 0.03479721316368587780, 0.03636223656666148080 ),
 .UNSPECIFIED. ) ;
#15637=FACE_OUTER_BOUND ( 'NONE', #5718, .T. ) ;
#15638=DIRECTION ( 'NONE',  ( 0.000000000000000000, 0.000000000000000000, 1.000000000000000000 ) ) ;
#15648=CARTESIAN_POINT ( 'NONE',  ( 20.42502041961813930, 230.5765313837437418, 60.00000000000000000 ) ) ;
#15653=CARTESIAN_POINT ( 'NONE',  ( 43.53705524234220547, 56.85652257517428865, -96.62835994548002816 ) ) ;
#15659=ORIENTED_EDGE ( 'NONE', *, *, #1809, .F. ) ;
#15661=ORIENTED_EDGE ( 'NONE', *, *, #15458, .F. ) ;
#15667=CIRCLE ( 'NONE', #3895, 21.20245194746113526 ) ;
#15668=ORIENTED_EDGE ( 'NONE', *, *, #3720, .T. ) ;
#15679=DIRECTION ( 'NONE',  ( 0.000000000000000000, 0.000000000000000000, 1.000000000000000000 ) ) ;
#15681=CIRCLE ( 'NONE', #2550, 220.7252770684331438 ) ;
#15685=VERTEX_POINT ( 'NONE', #19889 ) ;
#15688=ORIENTED_EDGE ( 'NONE', *, *, #21318, .F. ) ;
#15691=ORIENTED_EDGE ( 'NONE', *, *, #14401, .F. ) ;
#15696=AXIS2_PLACEMENT_3D ( 'NONE', #2931, #7778, #3248 ) ;
#15710=CARTESIAN_POINT ( 'NONE',  ( 40.42502041961814996, 170.1716627696692683, -40.00000000000000000 ) ) ;
#15711=VERTEX_POINT ( 'NONE', #8920 ) ;
#15717=EDGE_CURVE ( 'NONE', #16350, #12966, #2448, .T. ) ;
#15725=FACE_OUTER_BOUND ( 'NONE', #9569, .T. ) ;
#15737=VERTEX_POINT ( 'NONE', #12285 ) ;
#15744=FACE_OUTER_BOUND ( 'NONE', #7553, .T. ) ;
#15754=DIRECTION ( 'NONE',  ( -0.02283316540262222277, 0.9997392892938120612, 0.000000000000000000 ) ) ;
#15755=LINE ( 'NONE', #4280, #7665 ) ;
#15756=LINE ( 'NONE', #18556, #20079 ) ;
#15763=ORIENTED_EDGE ( 'NONE', *, *, #12390, .F. ) ;
#15774=AXIS2_PLACEMENT_3D ( 'NONE', #7480, #1229, #2742 ) ;
#15777=ADVANCED_FACE ( 'NONE', ( #17467, #4594 ), #19305, .T. ) ;
#15778=DIRECTION ( 'NONE',  ( 0.000000000000000000, 0.000000000000000000, 1.000000000000000000 ) ) ;
#15781=VECTOR ( 'NONE', #11592, 1000.000000000000000 ) ;
#15783=DIRECTION ( 'NONE',  ( 0.9997392892938121722, 0.02283316540262222971, -0.000000000000000000 ) ) ;
#15786=CARTESIAN_POINT ( 'NONE',  ( 29.72350413846044859, 280.4463447002762564, 40.00000000000000000 ) ) ;
#15788=VECTOR ( 'NONE', #14775, 1000.000000000000114 ) ;
#15792=ADVANCED_FACE ( 'NONE', ( #14558 ), #12713, .T. ) ;
#15793=VECTOR ( 'NONE', #2657, 1000.000000000000000 ) ;
#15797=ORIENTED_EDGE ( 'NONE', *, *, #4148, .T. ) ;
#15800=VERTEX_POINT ( 'NONE', #12503 ) ;
#15802=ORIENTED_EDGE ( 'NONE', *, *, #10096, .F. ) ;
#15805=AXIS2_PLACEMENT_3D ( 'NONE', #5039, #14691, #13383 ) ;
#15811=EDGE_CURVE ( 'NONE', #17379, #1316, #17369, .T. ) ;
#15813=DIRECTION ( 'NONE',  ( 0.000000000000000000, 0.000000000000000000, -1.000000000000000000 ) ) ;
#15817=VERTEX_POINT ( 'NONE', #15966 ) ;
#15819=AXIS2_PLACEMENT_3D ( 'NONE', #3296, #14982, #16283 ) ;
#15822=VERTEX_POINT ( 'NONE', #12821 ) ;
#15835=DIRECTION ( 'NONE',  ( -0.000000000000000000, 1.000000000000000000, -0.000000000000000000 ) ) ;
#15837=CARTESIAN_POINT ( 'NONE',  ( 65.85920792673738333, 170.1716627696692683, -40.00000000000000000 ) ) ;
#15845=VERTEX_POINT ( 'NONE', #12610 ) ;
#15848=VECTOR ( 'NONE', #14567, 1000.000000000000114 ) ;
#15849=EDGE_CURVE ( 'NONE', #17635, #8154, #19412, .T. ) ;
#15858=PRODUCT_DEFINITION ( 'UNKNOWN', '', #15588, #785 ) ;
#15862=DIRECTION ( 'NONE',  ( 0.000000000000000000, -1.000000000000000000, 0.000000000000000000 ) ) ;
#15864=CIRCLE ( 'NONE', #21023, 59.93977357075245038 ) ;
#15871=ORIENTED_EDGE ( 'NONE', *, *, #10107, .F. ) ;
#15880=DIRECTION ( 'NONE',  ( 0.000000000000000000, 0.000000000000000000, 1.000000000000000000 ) ) ;
#15881=AXIS2_PLACEMENT_3D ( 'NONE', #10834, #5750, #1019 ) ;
#15892=EDGE_CURVE ( 'NONE', #2298, #1002, #14133, .T. ) ;
#15897=CARTESIAN_POINT ( 'NONE',  ( -162.2727221670389781, 30.52886280891152282, -20.57735571454641033 ) ) ;
#15904=VERTEX_POINT ( 'NONE', #20717 ) ;
#15910=EDGE_CURVE ( 'NONE', #19163, #10104, #8525, .T. ) ;
#15913=CIRCLE ( 'NONE', #26, 10.00000000000000533 ) ;
#15921=CARTESIAN_POINT ( 'NONE',  ( 6.416697501590670427, 217.7548513357008630, -60.00000000000000000 ) ) ;
#15923=EDGE_CURVE ( 'NONE', #16030, #5025, #19202, .T. ) ;
#15925=AXIS2_PLACEMENT_3D ( 'NONE', #16731, #5452, #1918 ) ;
#15940=LINE ( 'NONE', #6391, #10040 ) ;
#15942=AXIS2_PLACEMENT_3D ( 'NONE', #17265, #10435, #12066 ) ;
#15949=EDGE_LOOP ( 'NONE', ( #6586, #15802 ) ) ;
#15950=DIRECTION ( 'NONE',  ( -0.000000000000000000, -0.000000000000000000, -1.000000000000000000 ) ) ;
#15955=DIRECTION ( 'NONE',  ( -0.000000000000000000, -0.000000000000000000, -1.000000000000000000 ) ) ;
#15961=LINE ( 'NONE', #7398, #6175 ) ;
#15962=( GEOMETRIC_REPRESENTATION_CONTEXT ( 3 ) GLOBAL_UNCERTAINTY_ASSIGNED_CONTEXT ( ( #14829 ) ) GLOBAL_UNIT_ASSIGNED_CONTEXT ( ( #16111, #17721, #4953 ) ) REPRESENTATION_CONTEXT ( 'NONE', 'WORKASPACE' ) );
#15965=CARTESIAN_POINT ( 'NONE',  ( 164.2593879927715932, 166.6963511708817691, -60.00000000000000000 ) ) ;
#15966=CARTESIAN_POINT ( 'NONE',  ( 78.68120802659203150, 149.7457237375499517, 66.14548919766383506 ) ) ;
#15969=ADVANCED_FACE ( 'NONE', ( #6100 ), #19095, .F. ) ;
#15977=VERTEX_POINT ( 'NONE', #7826 ) ;
#15990=LINE ( 'NONE', #7312, #9359 ) ;
#16003=DIRECTION ( 'NONE',  ( 0.000000000000000000, 0.000000000000000000, 1.000000000000000000 ) ) ;
#16007=CIRCLE ( 'NONE', #6318, 4.000000000000001776 ) ;
#16010=EDGE_LOOP ( 'NONE', ( #5905, #2060, #18778, #15389 ) ) ;
#16013=FACE_OUTER_BOUND ( 'NONE', #402, .T. ) ;
#16019=FACE_OUTER_BOUND ( 'NONE', #8956, .T. ) ;
#16027=DIRECTION ( 'NONE',  ( -0.000000000000000000, -0.000000000000000000, -1.000000000000000000 ) ) ;
#16030=VERTEX_POINT ( 'NONE', #19516 ) ;
#16031=EDGE_LOOP ( 'NONE', ( #6141, #16967, #12346 ) ) ;
#16038=EDGE_CURVE ( 'NONE', #880, #12697, #1904, .T. ) ;
#16040=DIRECTION ( 'NONE',  ( 1.000000000000000000, 0.000000000000000000, 0.000000000000000000 ) ) ;
#16046=DIRECTION ( 'NONE',  ( 1.000000000000000000, 0.000000000000000000, 0.000000000000000000 ) ) ;
#16050=DIRECTION ( 'NONE',  ( -0.000000000000000000, -0.000000000000000000, 1.000000000000000000 ) ) ;
#16064=CYLINDRICAL_SURFACE ( 'NONE', #11075, 20.00000000000000000 ) ;
#16072=CARTESIAN_POINT ( 'NONE',  ( 51.98467606588575052, 30.52886280891152282, -117.7257097687431298 ) ) ;
#16079=ORIENTED_EDGE ( 'NONE', *, *, #19266, .T. ) ;
#16081=VERTEX_POINT ( 'NONE', #16288 ) ;
#16084=EDGE_LOOP ( 'NONE', ( #15606, #14091, #18914, #18508 ) ) ;
#16087=VERTEX_POINT ( 'NONE', #14670 ) ;
#16089=CARTESIAN_POINT ( 'NONE',  ( 72.94945500224395118, 285.0140030772282103, 20.00000000000000355 ) ) ;
#16092=CARTESIAN_POINT ( 'NONE',  ( 10.41669750159067220, 217.7548513357008630, -49.99999999999999289 ) ) ;
#16102=EDGE_CURVE ( 'NONE', #12697, #7658, #18318, .T. ) ;
#16104=EDGE_CURVE ( 'NONE', #2702, #604, #11508, .T. ) ;
#16109=VERTEX_POINT ( 'NONE', #5126 ) ;
#16111=( LENGTH_UNIT ( ) NAMED_UNIT ( * ) SI_UNIT ( .MILLI., .METRE. ) );
#16113=ORIENTED_EDGE ( 'NONE', *, *, #17082, .F. ) ;
#16122=CIRCLE ( 'NONE', #18868, 49.93977357075243617 ) ;
#16128=CARTESIAN_POINT ( 'NONE',  ( 30.42502041961814996, 180.1716627696692967, -40.00000000000000000 ) ) ;
#16132=ORIENTED_EDGE ( 'NONE', *, *, #8147, .F. ) ;
#16133=ORIENTED_EDGE ( 'NONE', *, *, #5051, .T. ) ;
#16153=AXIS2_PLACEMENT_3D ( 'NONE', #3400, #19944, #19724 ) ;
#16161=VERTEX_POINT ( 'NONE', #14770 ) ;
#16162=LINE ( 'NONE', #1553, #7396 ) ;
#16167=DIRECTION ( 'NONE',  ( -0.000000000000000000, -0.000000000000000000, 1.000000000000000000 ) ) ;
#16169=ORIENTED_EDGE ( 'NONE', *, *, #21038, .T. ) ;
#16171=DIRECTION ( 'NONE',  ( -3.836511174089486666E-16, 0.000000000000000000, -1.000000000000000000 ) ) ;
#16178=DIRECTION ( 'NONE',  ( -0.000000000000000000, 1.000000000000000000, 0.000000000000000000 ) ) ;
#16188=ORIENTED_EDGE ( 'NONE', *, *, #10326, .T. ) ;
#16192=DIRECTION ( 'NONE',  ( 1.000000000000000000, 0.000000000000000000, 0.000000000000000000 ) ) ;
#16196=CARTESIAN_POINT ( 'NONE',  ( -123.2946569474810303, 30.52886280891152282, -20.57735571454641388 ) ) ;
#16199=DIRECTION ( 'NONE',  ( 0.000000000000000000, 1.000000000000000000, 0.000000000000000000 ) ) ;
#16210=DIRECTION ( 'NONE',  ( 0.000000000000000000, 1.000000000000000000, 0.000000000000000000 ) ) ;
#16215=AXIS2_PLACEMENT_3D ( 'NONE', #8357, #14981, #168 ) ;
#16217=ORIENTED_EDGE ( 'NONE', *, *, #10816, .T. ) ;
#16221=ORIENTED_EDGE ( 'NONE', *, *, #7005, .T. ) ;
#16230=AXIS2_PLACEMENT_3D ( 'NONE', #12114, #18284, #8439 ) ;
#16233=ADVANCED_FACE ( 'NONE', ( #9984 ), #18210, .F. ) ;
#16235=EDGE_CURVE ( 'NONE', #1858, #10342, #174, .T. ) ;
#16241=ORIENTED_EDGE ( 'NONE', *, *, #4063, .T. ) ;
#16242=ORIENTED_EDGE ( 'NONE', *, *, #17683, .F. ) ;
#16249=DIRECTION ( 'NONE',  ( 0.000000000000000000, 0.000000000000000000, -1.000000000000000000 ) ) ;
#16255=VECTOR ( 'NONE', #12165, 1000.000000000000000 ) ;
#16256=CIRCLE ( 'NONE', #10111, 22.72497359561857877 ) ;
#16268=VECTOR ( 'NONE', #15950, 1000.000000000000000 ) ;
#16271=CARTESIAN_POINT ( 'NONE',  ( 0.000000000000000000, 56.85652257517428865, 0.000000000000000000 ) ) ;
#16274=CARTESIAN_POINT ( 'NONE',  ( -22.30770786884145451, 10.52886280891152104, -122.9933582338429972 ) ) ;
#16279=DIRECTION ( 'NONE',  ( 0.000000000000000000, 1.000000000000000000, 0.000000000000000000 ) ) ;
#16282=CARTESIAN_POINT ( 'NONE',  ( -28.46624702801777573, 47.09320012170705638, 49.60091809715360256 ) ) ;
#16283=DIRECTION ( 'NONE',  ( 0.1337298367054296222, -0.9910178256594273094, 0.000000000000000000 ) ) ;
#16288=CARTESIAN_POINT ( 'NONE',  ( 20.42502041961806825, 281.1055109169419666, -40.00000000000000000 ) ) ;
#16289=VECTOR ( 'NONE', #18319, 1000.000000000000000 ) ;
#16291=EDGE_CURVE ( 'NONE', #20443, #17320, #6105, .T. ) ;
#16292=CARTESIAN_POINT ( 'NONE',  ( -18.68588794268873698, 323.8848358243226357, -20.00000000000000355 ) ) ;
#16298=ORIENTED_EDGE ( 'NONE', *, *, #1499, .T. ) ;
#16301=ORIENTED_EDGE ( 'NONE', *, *, #20255, .T. ) ;
#16302=VECTOR ( 'NONE', #5822, 1000.000000000000000 ) ;
#16329=ORIENTED_EDGE ( 'NONE', *, *, #19782, .F. ) ;
#16339=CARTESIAN_POINT ( 'NONE',  ( 91.21585410611801592, 56.85652257517428865, 94.99999999999994316 ) ) ;
#16345=VERTEX_POINT ( 'NONE', #13577 ) ;
#16348=ORIENTED_EDGE ( 'NONE', *, *, #10400, .T. ) ;
#16349=ORIENTED_EDGE ( 'NONE', *, *, #18779, .F. ) ;
#16350=VERTEX_POINT ( 'NONE', #494 ) ;
#16361=CARTESIAN_POINT ( 'NONE',  ( 6.416697501590670427, 172.9933428177121471, -60.00000000000000000 ) ) ;
#16364=CARTESIAN_POINT ( 'NONE',  ( 0.000000000000000000, 0.000000000000000000, 40.00000000000000000 ) ) ;
#16368=VECTOR ( 'NONE', #13180, 1000.000000000000000 ) ;
#16377=ORIENTED_EDGE ( 'NONE', *, *, #13066, .F. ) ;
#16380=CARTESIAN_POINT ( 'NONE',  ( -30.19626789828514646, 48.38008749069921777, 49.58203932211407761 ) ) ;
#16387=ADVANCED_FACE ( 'NONE', ( #698 ), #20057, .F. ) ;
#16389=LINE ( 'NONE', #1790, #2391 ) ;
#16391=CARTESIAN_POINT ( 'NONE',  ( 65.85920792673738333, 160.1716627696692683, -40.00000000000000000 ) ) ;
#16392=LINE ( 'NONE', #19304, #3217 ) ;
#16393=AXIS2_PLACEMENT_3D ( 'NONE', #9692, #13056, #11103 ) ;
#16401=VERTEX_POINT ( 'NONE', #385 ) ;
#16409=ORIENTED_EDGE ( 'NONE', *, *, #14921, .F. ) ;
#16411=LINE ( 'NONE', #3209, #19028 ) ;
#16418=CARTESIAN_POINT ( 'NONE',  ( 0.000000000000000000, 31.85652257517428865, 0.000000000000000000 ) ) ;
#16423=CYLINDRICAL_SURFACE ( 'NONE', #9200, 49.93977357075243617 ) ;
#16425=EDGE_CURVE ( 'NONE', #15077, #16081, #13675, .T. ) ;
#16429=VERTEX_POINT ( 'NONE', #17027 ) ;
#16431=EDGE_CURVE ( 'NONE', #763, #7305, #7267, .T. ) ;
#16438=DIRECTION ( 'NONE',  ( 1.232945044042657126E-32, -9.855701800883825964E-17, 1.000000000000000000 ) ) ;
#16448=DIRECTION ( 'NONE',  ( -1.000000000000000000, 0.000000000000000000, 0.000000000000000000 ) ) ;
#16449=ORIENTED_EDGE ( 'NONE', *, *, #18119, .F. ) ;
#16457=DIRECTION ( 'NONE',  ( 1.000000000000000000, 0.000000000000000000, -0.000000000000000000 ) ) ;
#16463=EDGE_CURVE ( 'NONE', #14441, #9372, #12790, .T. ) ;
#16471=CARTESIAN_POINT ( 'NONE',  ( 20.42502041961813575, 271.1055109169419666, 40.00000000000000000 ) ) ;
#16491=CARTESIAN_POINT ( 'NONE',  ( 51.98438129372387806, 30.52886280891151216, -117.7249735956185219 ) ) ;
#16493=CARTESIAN_POINT ( 'NONE',  ( -17.27065617357490268, 46.46077788388278407, 48.27172322967895468 ) ) ;
#16495=DIRECTION ( 'NONE',  ( 0.000000000000000000, 0.000000000000000000, 1.000000000000000000 ) ) ;
#16498=AXIS2_PLACEMENT_3D ( 'NONE', #1149, #7720, #17573 ) ;
#16500=LINE ( 'NONE', #13141, #3109 ) ;
#16502=VECTOR ( 'NONE', #9187, 1000.000000000000000 ) ;
#16509=DIRECTION ( 'NONE',  ( 3.836511174089486666E-16, 0.000000000000000000, -1.000000000000000000 ) ) ;
#16510=EDGE_LOOP ( 'NONE', ( #10522, #20848, #17113, #13012 ) ) ;
#16513=EDGE_LOOP ( 'NONE', ( #3171, #12936 ) ) ;
#16528=LINE ( 'NONE', #94, #16812 ) ;
#16535=ORIENTED_EDGE ( 'NONE', *, *, #11869, .T. ) ;
#16546=DIRECTION ( 'NONE',  ( 3.836511174089486173E-16, -0.000000000000000000, 1.000000000000000000 ) ) ;
#16550=DIRECTION ( 'NONE',  ( 0.000000000000000000, -1.000000000000000000, 0.000000000000000000 ) ) ;
#16551=EDGE_CURVE ( 'NONE', #2936, #13, #1126, .T. ) ;
#16558=VERTEX_POINT ( 'NONE', #1022 ) ;
#16560=VERTEX_POINT ( 'NONE', #10940 ) ;
#16561=ORIENTED_EDGE ( 'NONE', *, *, #10537, .T. ) ;
#16571=EDGE_CURVE ( 'NONE', #14089, #11949, #7488, .T. ) ;
#16577=CARTESIAN_POINT ( 'NONE',  ( -28.68588794268872277, 250.8848358243226357, -20.00000000000000000 ) ) ;
#16583=ORIENTED_EDGE ( 'NONE', *, *, #18034, .T. ) ;
#16586=AXIS2_PLACEMENT_3D ( 'NONE', #13302, #5174, #10349 ) ;
#16588=DIRECTION ( 'NONE',  ( -9.855701800883827197E-17, 1.000000000000000000, 0.000000000000000000 ) ) ;
#16601=CARTESIAN_POINT ( 'NONE',  ( -28.68588794268872633, 250.8848358243226357, 0.000000000000000000 ) ) ;
#16607=CARTESIAN_POINT ( 'NONE',  ( -28.68588794268874054, 271.1055109169419666, 40.00000000000000000 ) ) ;
#16611=CARTESIAN_POINT ( 'NONE',  ( -23.06691706883066928, 45.31613216062292082, -122.8556579767893027 ) ) ;
#16616=EDGE_LOOP ( 'NONE', ( #5690, #4426, #8771, #7741, #19898 ) ) ;
#16620=ORIENTED_EDGE ( 'NONE', *, *, #1382, .F. ) ;
#16623=VERTEX_POINT ( 'NONE', #17656 ) ;
#16625=CARTESIAN_POINT ( 'NONE',  ( -23.82844689576343100, 45.41375816275737520, -49.36319628876446330 ) ) ;
#16628=VECTOR ( 'NONE', #5097, 1000.000000000000000 ) ;
#16629=CARTESIAN_POINT ( 'NONE',  ( -28.68588794268872633, 250.8848358243226357, 20.00000000000000000 ) ) ;
#16632=CYLINDRICAL_SURFACE ( 'NONE', #11476, 4.000000000000001776 ) ;
#16635=CARTESIAN_POINT ( 'NONE',  ( 60.03793209889851568, 30.52886280891152282, -136.1729372809869005 ) ) ;
#16639=DIRECTION ( 'NONE',  ( -0.000000000000000000, -0.000000000000000000, -1.000000000000000000 ) ) ;
#16641=CARTESIAN_POINT ( 'NONE',  ( -29.07862423524327156, 47.49931253676632537, -49.60091809715360256 ) ) ;
#16643=EDGE_CURVE ( 'NONE', #5454, #16087, #18953, .T. ) ;
#16647=EDGE_CURVE ( 'NONE', #5288, #13870, #4991, .T. ) ;
#16650=ORIENTED_EDGE ( 'NONE', *, *, #9568, .F. ) ;
#16654=ORIENTED_EDGE ( 'NONE', *, *, #12536, .F. ) ;
#16655=CARTESIAN_POINT ( 'NONE',  ( 125.7989814974898053, 10.52886280891152104, -40.00000000000000000 ) ) ;
#16667=DIRECTION ( 'NONE',  ( 0.000000000000000000, 0.000000000000000000, 1.000000000000000000 ) ) ;
#16670=ORIENTED_EDGE ( 'NONE', *, *, #4468, .T. ) ;
#16681=LINE ( 'NONE', #11693, #3101 ) ;
#16684=AXIS2_PLACEMENT_3D ( 'NONE', #21141, #19514, #3078 ) ;
#16689=CARTESIAN_POINT ( 'NONE',  ( 60.03793209889851568, 10.52886280891152104, -126.1729372809868863 ) ) ;
#16712=DIRECTION ( 'NONE',  ( 0.000000000000000000, -1.000000000000000000, 0.000000000000000000 ) ) ;
#16715=AXIS2_PLACEMENT_3D ( 'NONE', #7656, #19238, #2806 ) ;
#16718=VECTOR ( 'NONE', #9766, 1000.000000000000000 ) ;
#16730=VERTEX_POINT ( 'NONE', #16577 ) ;
#16731=CARTESIAN_POINT ( 'NONE',  ( 60.03793209889851568, 10.52886280891152104, 131.1729372809869005 ) ) ;
#16735=CARTESIAN_POINT ( 'NONE',  ( -24.85718862968342435, 45.58919278729139535, -49.45561310859971371 ) ) ;
#16739=CYLINDRICAL_SURFACE ( 'NONE', #13042, 4.000000000000001776 ) ;
#16740=CARTESIAN_POINT ( 'NONE',  ( 78.68120802659204571, 149.7457237375499517, -20.00000000000000355 ) ) ;
#16743=DIRECTION ( 'NONE',  ( 1.000000000000000000, 0.000000000000000000, -0.000000000000000000 ) ) ;
#16751=ORIENTED_EDGE ( 'NONE', *, *, #18350, .T. ) ;
#16752=CARTESIAN_POINT ( 'NONE',  ( -22.30770786884145451, 30.52886280891152282, 122.9933582338429972 ) ) ;
#16771=EDGE_LOOP ( 'NONE', ( #15668, #11780 ) ) ;
#16786=CYLINDRICAL_SURFACE ( 'NONE', #16230, 22.72497359561857877 ) ;
#16788=DIRECTION ( 'NONE',  ( 0.000000000000000000, -0.000000000000000000, 1.000000000000000000 ) ) ;
#16802=DIRECTION ( 'NONE',  ( -1.250996701150283068E-16, 1.000000000000000000, 0.000000000000000000 ) ) ;
#16805=CARTESIAN_POINT ( 'NONE',  ( -123.2946569474810019, 30.52886280891154058, -20.57735571454641388 ) ) ;
#16811=CARTESIAN_POINT ( 'NONE',  ( 60.03793209889851568, 30.52886280891152282, 131.1729372809869005 ) ) ;
#16812=VECTOR ( 'NONE', #20090, 1000.000000000000000 ) ;
#16817=LINE ( 'NONE', #20054, #6571 ) ;
#16821=CIRCLE ( 'NONE', #11958, 210.7252770684331438 ) ;
#16823=CARTESIAN_POINT ( 'NONE',  ( -28.68588794268873698, -129.7637193493918915, 0.000000000000000000 ) ) ;
#16824=EDGE_CURVE ( 'NONE', #3730, #9937, #2011, .T. ) ;
#16832=ORIENTED_EDGE ( 'NONE', *, *, #5370, .F. ) ;
#16837=CARTESIAN_POINT ( 'NONE',  ( -28.25075301531890304, 46.95029017519802750, -49.60091809715360966 ) ) ;
#16840=LINE ( 'NONE', #15330, #14827 ) ;
#16843=FACE_OUTER_BOUND ( 'NONE', #10048, .T. ) ;
#16849=DIRECTION ( 'NONE',  ( 0.000000000000000000, 0.000000000000000000, -1.000000000000000000 ) ) ;
#16856=EDGE_CURVE ( 'NONE', #15800, #11839, #15255, .T. ) ;
#16860=CARTESIAN_POINT ( 'NONE',  ( 43.53705524234220547, 56.85652257517428865, -96.62835994548002816 ) ) ;
#16866=ADVANCED_FACE ( 'NONE', ( #10379 ), #18498, .T. ) ;
#16868=DIRECTION ( 'NONE',  ( 1.000000000000000000, 0.000000000000000000, 0.000000000000000000 ) ) ;
#16881=DIRECTION ( 'NONE',  ( 1.000000000000000000, 0.000000000000000000, 0.000000000000000000 ) ) ;
#16883=ORIENTED_EDGE ( 'NONE', *, *, #107, .F. ) ;
#16887=FACE_OUTER_BOUND ( 'NONE', #21074, .T. ) ;
#16904=CARTESIAN_POINT ( 'NONE',  ( -49.57497958038184294, -6.743947802724785386E-15, 0.000000000000000000 ) ) ;
#16905=ORIENTED_EDGE ( 'NONE', *, *, #4468, .F. ) ;
#16919=VECTOR ( 'NONE', #4483, 1000.000000000000000 ) ;
#16926=CARTESIAN_POINT ( 'NONE',  ( 30.42502041961813575, 271.1055109169419097, 20.00000000000000355 ) ) ;
#16927=CIRCLE ( 'NONE', #3781, 4.000000000000003553 ) ;
#16936=ORIENTED_EDGE ( 'NONE', *, *, #17946, .F. ) ;
#16941=DIRECTION ( 'NONE',  ( 0.000000000000000000, -1.000000000000000000, 0.000000000000000000 ) ) ;
#16945=LINE ( 'NONE', #14025, #3712 ) ;
#16961=AXIS2_PLACEMENT_3D ( 'NONE', #9541, #3062, #6506 ) ;
#16962=VERTEX_POINT ( 'NONE', #8653 ) ;
#16964=DIRECTION ( 'NONE',  ( 0.000000000000000000, 0.000000000000000000, -1.000000000000000000 ) ) ;
#16966=CIRCLE ( 'NONE', #7952, 22.72497359561857877 ) ;
#16967=ORIENTED_EDGE ( 'NONE', *, *, #15811, .F. ) ;
#16968=PLANE ( 'NONE',  #9709 ) ;
#16984=ORIENTED_EDGE ( 'NONE', *, *, #9663, .F. ) ;
#16986=ORIENTED_EDGE ( 'NONE', *, *, #14743, .F. ) ;
#17001=CARTESIAN_POINT ( 'NONE',  ( 28.16023193154655502, 323.8848358243226357, -20.00000000000000355 ) ) ;
#17003=DIRECTION ( 'NONE',  ( -1.232945044042657126E-32, 9.855701800883825964E-17, 1.000000000000000000 ) ) ;
#17006=ORIENTED_EDGE ( 'NONE', *, *, #15910, .T. ) ;
#17022=DIRECTION ( 'NONE',  ( -0.000000000000000000, 1.000000000000000000, -0.000000000000000000 ) ) ;
#17024=( NAMED_UNIT ( * ) SI_UNIT ( $, .STERADIAN. ) SOLID_ANGLE_UNIT ( ) );
#17027=CARTESIAN_POINT ( 'NONE',  ( 20.42502041961813930, 230.5765313837437418, -49.99999999999999289 ) ) ;
#17028=LINE ( 'NONE', #5544, #20773 ) ;
#17029=LINE ( 'NONE', #8795, #1972 ) ;
#17036=EDGE_LOOP ( 'NONE', ( #12266, #230, #5142, #17119 ) ) ;
#17041=CARTESIAN_POINT ( 'NONE',  ( -22.30770786884143675, 45.31613216062291372, 122.9933582338429687 ) ) ;
#17048=DIRECTION ( 'NONE',  ( -0.000000000000000000, -0.000000000000000000, 1.000000000000000000 ) ) ;
#17052=DIRECTION ( 'NONE',  ( 0.000000000000000000, 1.000000000000000000, 0.000000000000000000 ) ) ;
#17053=CARTESIAN_POINT ( 'NONE',  ( 52.60622592008805043, 30.52886280891152282, 151.0302712373927250 ) ) ;
#17070=CARTESIAN_POINT ( 'NONE',  ( 91.21585410611801592, 31.85652257517428865, -40.00000000000000000 ) ) ;
#17072=ORIENTED_EDGE ( 'NONE', *, *, #9208, .T. ) ;
#17073=DIRECTION ( 'NONE',  ( -1.000000000000000000, 0.000000000000000000, -0.000000000000000000 ) ) ;
#17082=EDGE_CURVE ( 'NONE', #12542, #13817, #19953, .T. ) ;
#17083=DIRECTION ( 'NONE',  ( 0.000000000000000000, -1.000000000000000000, 0.000000000000000000 ) ) ;
#17085=EDGE_CURVE ( 'NONE', #5504, #5552, #4108, .T. ) ;
#17086=PLANE ( 'NONE',  #12927 ) ;
#17089=FACE_OUTER_BOUND ( 'NONE', #4235, .T. ) ;
#17094=DIRECTION ( 'NONE',  ( 0.000000000000000000, 0.000000000000000000, -1.000000000000000000 ) ) ;
#17098=ORIENTED_EDGE ( 'NONE', *, *, #15442, .T. ) ;
#17107=EDGE_CURVE ( 'NONE', #12773, #2298, #889, .T. ) ;
#17113=ORIENTED_EDGE ( 'NONE', *, *, #6050, .T. ) ;
#17116=ORIENTED_EDGE ( 'NONE', *, *, #13966, .T. ) ;
#17119=ORIENTED_EDGE ( 'NONE', *, *, #11993, .T. ) ;
#17122=EDGE_CURVE ( 'NONE', #18169, #13, #15598, .T. ) ;
#17139=CARTESIAN_POINT ( 'NONE',  ( -32.80098538532548957, 52.03835429381459221, -120.6197264542505536 ) ) ;
#17144=ORIENTED_EDGE ( 'NONE', *, *, #6057, .T. ) ;
#17146=LINE ( 'NONE', #10524, #3238 ) ;
#17148=CARTESIAN_POINT ( 'NONE',  ( 0.000000000000000000, -343.0245277843623057, 0.000000000000000000 ) ) ;
#17154=CARTESIAN_POINT ( 'NONE',  ( 35.96497763894179656, 191.2380552923725645, -48.74187950074039577 ) ) ;
#17155=CARTESIAN_POINT ( 'NONE',  ( 118.4271928232701043, -343.0245277843623057, -40.00000000000000000 ) ) ;
#17158=VECTOR ( 'NONE', #13255, 1000.000000000000000 ) ;
#17160=CARTESIAN_POINT ( 'NONE',  ( -22.30770786884136214, -343.0245277843623057, 122.9933582338429972 ) ) ;
#17163=EDGE_CURVE ( 'NONE', #10333, #4398, #20664, .T. ) ;
#17168=DIRECTION ( 'NONE',  ( 0.000000000000000000, 0.000000000000000000, -1.000000000000000000 ) ) ;
#17189=AXIS2_PLACEMENT_3D ( 'NONE', #2234, #17052, #15538 ) ;
#17193=CARTESIAN_POINT ( 'NONE',  ( 51.50493485826542184, 141.8799693780962912, 94.99999999999994316 ) ) ;
#17195=VERTEX_POINT ( 'NONE', #7562 ) ;
#17197=ORIENTED_EDGE ( 'NONE', *, *, #13122, .T. ) ;
#17201=ORIENTED_EDGE ( 'NONE', *, *, #63, .T. ) ;
#17222=EDGE_LOOP ( 'NONE', ( #5162, #19788, #16241, #13585 ) ) ;
#17237=DIRECTION ( 'NONE',  ( 1.000000000000000000, 0.000000000000000000, 0.000000000000000000 ) ) ;
#17240=EDGE_CURVE ( 'NONE', #12430, #9807, #5784, .T. ) ;
#17246=ORIENTED_EDGE ( 'NONE', *, *, #11811, .T. ) ;
#17248=ORIENTED_EDGE ( 'NONE', *, *, #8963, .F. ) ;
#17255=ORIENTED_EDGE ( 'NONE', *, *, #8497, .F. ) ;
#17260=DIRECTION ( 'NONE',  ( 0.000000000000000000, 1.000000000000000000, 0.000000000000000000 ) ) ;
#17265=CARTESIAN_POINT ( 'NONE',  ( 30.42502041961813575, 271.1055109169419097, -20.00000000000000355 ) ) ;
#17273=ORIENTED_EDGE ( 'NONE', *, *, #2898, .T. ) ;
#17279=ADVANCED_FACE ( 'NONE', ( #4851 ), #19464, .F. ) ;
#17283=CARTESIAN_POINT ( 'NONE',  ( 51.50493485826542184, 160.1716627696692683, -61.61851857202071159 ) ) ;
#17284=AXIS2_PLACEMENT_3D ( 'NONE', #8909, #15422, #9231 ) ;
#17293=EDGE_CURVE ( 'NONE', #3575, #4551, #8087, .T. ) ;
#17304=EDGE_CURVE ( 'NONE', #18961, #5934, #18215, .T. ) ;
#17320=VERTEX_POINT ( 'NONE', #14824 ) ;
#17322=ORIENTED_EDGE ( 'NONE', *, *, #19528, .T. ) ;
#17327=AXIS2_PLACEMENT_3D ( 'NONE', #7765, #20976, #6144 ) ;
#17341=FACE_OUTER_BOUND ( 'NONE', #4652, .T. ) ;
#17353=ORIENTED_EDGE ( 'NONE', *, *, #8898, .T. ) ;
#17354=CARTESIAN_POINT ( 'NONE',  ( 60.03793209889851568, 30.52886280891152282, -131.1729372809869005 ) ) ;
#17356=DIRECTION ( 'NONE',  ( 0.000000000000000000, -1.000000000000000000, 0.000000000000000000 ) ) ;
#17357=DIRECTION ( 'NONE',  ( 0.000000000000000000, 0.000000000000000000, 1.000000000000000000 ) ) ;
#17359=VECTOR ( 'NONE', #9728, 1000.000000000000000 ) ;
#17360=EDGE_LOOP ( 'NONE', ( #14996, #19424, #11941, #5820 ) ) ;
#17362=FACE_OUTER_BOUND ( 'NONE', #15371, .T. ) ;
#17366=LINE ( 'NONE', #2653, #3366 ) ;
#17369=LINE ( 'NONE', #1356, #15793 ) ;
#17377=CARTESIAN_POINT ( 'NONE',  ( 35.96497763894178945, 170.1716627696692683, -20.00000000000000355 ) ) ;
#17379=VERTEX_POINT ( 'NONE', #16339 ) ;
#17381=VERTEX_POINT ( 'NONE', #6468 ) ;
#17386=VECTOR ( 'NONE', #4649, 1000.000000000000000 ) ;
#17387=EDGE_LOOP ( 'NONE', ( #20016, #3517, #10550, #12565, #3674, #8879 ) ) ;
#17389=DIRECTION ( 'NONE',  ( -0.000000000000000000, 1.000000000000000000, -0.000000000000000000 ) ) ;
#17392=DIRECTION ( 'NONE',  ( 0.000000000000000000, 0.000000000000000000, 1.000000000000000000 ) ) ;
#17393=LINE ( 'NONE', #6230, #21178 ) ;
#17400=VECTOR ( 'NONE', #14810, 1000.000000000000000 ) ;
#17403=VECTOR ( 'NONE', #13917, 1000.000000000000000 ) ;
#17407=EDGE_LOOP ( 'NONE', ( #20038, #20180, #19738, #7545, #8825, #17516 ) ) ;
#17424=CARTESIAN_POINT ( 'NONE',  ( -18.68588794268873698, 323.8848358243226357, 40.00000000000000000 ) ) ;
#17425=DIRECTION ( 'NONE',  ( -1.000000000000000000, -1.374938938973709817E-16, 0.000000000000000000 ) ) ;
#17432=VERTEX_POINT ( 'NONE', #4746 ) ;
#17433=CARTESIAN_POINT ( 'NONE',  ( -28.68588794268872277, 250.8848358243226357, -40.00000000000000000 ) ) ;
#17436=CARTESIAN_POINT ( 'NONE',  ( 91.21585410611801592, 31.85652257517428865, -40.00000000000000000 ) ) ;
#17446=CARTESIAN_POINT ( 'NONE',  ( 78.68120802659203150, 149.7457237375499517, 94.99999999999994316 ) ) ;
#17451=ORIENTED_EDGE ( 'NONE', *, *, #15071, .F. ) ;
#17453=ORIENTED_EDGE ( 'NONE', *, *, #17293, .T. ) ;
#17454=FACE_BOUND ( 'NONE', #3754, .T. ) ;
#17467=FACE_BOUND ( 'NONE', #10745, .T. ) ;
#17468=DIRECTION ( 'NONE',  ( -0.000000000000000000, -0.000000000000000000, 1.000000000000000000 ) ) ;
#17475=DIRECTION ( 'NONE',  ( 0.000000000000000000, -0.000000000000000000, -1.000000000000000000 ) ) ;
#17480=VERTEX_POINT ( 'NONE', #8628 ) ;
#17482=VERTEX_POINT ( 'NONE', #6794 ) ;
#17483=DIRECTION ( 'NONE',  ( 1.000000000000000000, 0.000000000000000000, 0.000000000000000000 ) ) ;
#17485=VERTEX_POINT ( 'NONE', #15363 ) ;
#17487=CARTESIAN_POINT ( 'NONE',  ( 51.98438129372387806, 30.52886280891151216, -94.99999999999994316 ) ) ;
#17489=CIRCLE ( 'NONE', #18174, 125.0000000000000000 ) ;
#17492=DIRECTION ( 'NONE',  ( 1.000000000000000000, 0.000000000000000000, 0.000000000000000000 ) ) ;
#17496=CYLINDRICAL_SURFACE ( 'NONE', #12167, 49.60091809715359545 ) ;
#17502=VECTOR ( 'NONE', #17168, 1000.000000000000000 ) ;
#17507=VERTEX_POINT ( 'NONE', #116 ) ;
#17512=CARTESIAN_POINT ( 'NONE',  ( 51.50493485826542184, 160.1716627696692683, 40.00000000000000000 ) ) ;
#17513=ORIENTED_EDGE ( 'NONE', *, *, #9276, .F. ) ;
#17516=ORIENTED_EDGE ( 'NONE', *, *, #17122, .F. ) ;
#17519=VECTOR ( 'NONE', #6764, 1000.000000000000000 ) ;
#17532=ORIENTED_EDGE ( 'NONE', *, *, #11425, .F. ) ;
#17533=ORIENTED_EDGE ( 'NONE', *, *, #6426, .T. ) ;
#17535=DIRECTION ( 'NONE',  ( 0.000000000000000000, 0.000000000000000000, -1.000000000000000000 ) ) ;
#17543=EDGE_CURVE ( 'NONE', #6011, #19571, #14793, .T. ) ;
#17545=EDGE_CURVE ( 'NONE', #9392, #15904, #13628, .T. ) ;
#17551=DIRECTION ( 'NONE',  ( -0.000000000000000000, 1.000000000000000000, -0.000000000000000000 ) ) ;
#17552=DIRECTION ( 'NONE',  ( 0.000000000000000000, 0.000000000000000000, -1.000000000000000000 ) ) ;
#17561=ORIENTED_EDGE ( 'NONE', *, *, #20302, .T. ) ;
#17562=CYLINDRICAL_SURFACE ( 'NONE', #13967, 5.000000000000004441 ) ;
#17573=DIRECTION ( 'NONE',  ( 0.000000000000000000, 0.000000000000000000, 1.000000000000000000 ) ) ;
#17574=LINE ( 'NONE', #15648, #12572 ) ;
#17575=DIRECTION ( 'NONE',  ( 1.000000000000000000, 0.000000000000000000, -0.000000000000000000 ) ) ;
#17590=VERTEX_POINT ( 'NONE', #18684 ) ;
#17593=ORIENTED_EDGE ( 'NONE', *, *, #4848, .F. ) ;
#17609=CIRCLE ( 'NONE', #16586, 125.0000000000000000 ) ;
#17614=DIRECTION ( 'NONE',  ( 1.000000000000000000, 0.000000000000000000, 0.000000000000000000 ) ) ;
#17626=CARTESIAN_POINT ( 'NONE',  ( -49.57497958038186425, 230.5765313837437418, -60.00000000000000000 ) ) ;
#17629=VECTOR ( 'NONE', #12625, 1000.000000000000114 ) ;
#17631=VECTOR ( 'NONE', #5559, 1000.000000000000000 ) ;
#17635=VERTEX_POINT ( 'NONE', #12640 ) ;
#17639=ORIENTED_EDGE ( 'NONE', *, *, #15892, .T. ) ;
#17640=DIRECTION ( 'NONE',  ( -0.000000000000000000, -0.000000000000000000, 1.000000000000000000 ) ) ;
#17644=VECTOR ( 'NONE', #19868, 1000.000000000000000 ) ;
#17649=CARTESIAN_POINT ( 'NONE',  ( 60.03793209889851568, 10.52886280891152104, -131.1729372809869005 ) ) ;
#17656=CARTESIAN_POINT ( 'NONE',  ( 30.42502041961814996, 180.1716627696692967, 20.00000000000000355 ) ) ;
#17659=AXIS2_PLACEMENT_3D ( 'NONE', #10541, #15435, #2342 ) ;
#17673=DIRECTION ( 'NONE',  ( 0.000000000000000000, -0.000000000000000000, 1.000000000000000000 ) ) ;
#17678=FACE_BOUND ( 'NONE', #15949, .T. ) ;
#17679=DIRECTION ( 'NONE',  ( 0.000000000000000000, 0.9253149302858357794, -0.3791995250394160633 ) ) ;
#17680=LINE ( 'NONE', #15965, #13923 ) ;
#17682=ADVANCED_FACE ( 'NONE', ( #5923 ), #13951, .F. ) ;
#17683=EDGE_CURVE ( 'NONE', #18164, #20120, #6420, .T. ) ;
#17690=EDGE_CURVE ( 'NONE', #19655, #9392, #7812, .T. ) ;
#17692=CARTESIAN_POINT ( 'NONE',  ( 60.69669829156632090, 56.85652257517428865, -94.99999999999994316 ) ) ;
#17704=CARTESIAN_POINT ( 'NONE',  ( 292.4526463419396691, 308.2087638784415162, -40.00000000000000000 ) ) ;
#17721=( NAMED_UNIT ( * ) PLANE_ANGLE_UNIT ( ) SI_UNIT ( $, .RADIAN. ) );
#17724=VERTEX_POINT ( 'NONE', #20539 ) ;
#17728=EDGE_CURVE ( 'NONE', #8877, #952, #12311, .T. ) ;
#17735=CARTESIAN_POINT ( 'NONE',  ( -18.68588794268873698, 281.1055109169419666, 20.00000000000000355 ) ) ;
#17744=EDGE_LOOP ( 'NONE', ( #14304, #8695, #602, #12326 ) ) ;
#17746=CARTESIAN_POINT ( 'NONE',  ( 10.41669750159067220, 217.7548513357008630, -60.00000000000000000 ) ) ;
#17749=AXIS2_PLACEMENT_3D ( 'NONE', #6157, #21204, #14410 ) ;
#17751=CARTESIAN_POINT ( 'NONE',  ( 116.0391604516428430, 192.9550247130592027, -40.00000000000000000 ) ) ;
#17756=EDGE_CURVE ( 'NONE', #2858, #9302, #7429, .T. ) ;
#17788=DIRECTION ( 'NONE',  ( -0.9365583756827543516, 0.000000000000000000, 0.3505116388060184329 ) ) ;
#17796=ORIENTED_EDGE ( 'NONE', *, *, #1583, .T. ) ;
#17808=DIRECTION ( 'NONE',  ( -0.000000000000000000, -1.000000000000000000, -0.000000000000000000 ) ) ;
#17812=DIRECTION ( 'NONE',  ( 0.000000000000000000, 0.000000000000000000, 1.000000000000000000 ) ) ;
#17814=DIRECTION ( 'NONE',  ( 0.1238475123623134638, -0.9177839099959486102, 0.3772724323803887114 ) ) ;
#17825=LINE ( 'NONE', #12964, #5584 ) ;
#17831=LINE ( 'NONE', #4643, #11728 ) ;
#17840=ORIENTED_EDGE ( 'NONE', *, *, #17163, .T. ) ;
#17842=ORIENTED_EDGE ( 'NONE', *, *, #14580, .T. ) ;
#17857=DIRECTION ( 'NONE',  ( 0.9365583756827543516, -0.000000000000000000, -0.3505116388060184329 ) ) ;
#17860=DIRECTION ( 'NONE',  ( 0.000000000000000000, 0.000000000000000000, 1.000000000000000000 ) ) ;
#17863=CIRCLE ( 'NONE', #15805, 10.00000000000000178 ) ;
#17868=EDGE_CURVE ( 'NONE', #11758, #12542, #12956, .T. ) ;
#17871=CARTESIAN_POINT ( 'NONE',  ( 91.21585410611801592, 56.85652257517428865, 94.99999999999994316 ) ) ;
#17874=CARTESIAN_POINT ( 'NONE',  ( 60.74769842942832554, 56.85652257517428865, 40.00000000000000000 ) ) ;
#17880=CYLINDRICAL_SURFACE ( 'NONE', #5184, 9.999999999999994671 ) ;
#17884=CARTESIAN_POINT ( 'NONE',  ( 88.28695088269886071, 142.5259582928263455, -40.00000000000000000 ) ) ;
#17889=DIRECTION ( 'NONE',  ( -0.000000000000000000, -0.000000000000000000, -1.000000000000000000 ) ) ;
#17892=FACE_OUTER_BOUND ( 'NONE', #6646, .T. ) ;
#17894=EDGE_CURVE ( 'NONE', #795, #12450, #11426, .T. ) ;
#17903=ORIENTED_EDGE ( 'NONE', *, *, #10809, .F. ) ;
#17905=DIRECTION ( 'NONE',  ( 0.02112707654195870172, -0.9250389998264586522, -0.3792841882241536067 ) ) ;
#17911=LINE ( 'NONE', #1381, #8417 ) ;
#17924=ORIENTED_EDGE ( 'NONE', *, *, #3873, .F. ) ;
#17926=CARTESIAN_POINT ( 'NONE',  ( -49.57497958038186425, 230.5765313837437418, -49.99999999999999289 ) ) ;
#17930=AXIS2_PLACEMENT_3D ( 'NONE', #1816, #16941, #15216 ) ;
#17934=CARTESIAN_POINT ( 'NONE',  ( 6.416697501590670427, 217.7548513357008630, -49.99999999999999289 ) ) ;
#17938=EDGE_CURVE ( 'NONE', #8292, #6060, #8148, .T. ) ;
#17941=CARTESIAN_POINT ( 'NONE',  ( -162.2727221670389781, 30.52886280891152282, 20.57735571454641033 ) ) ;
#17943=PLANE ( 'NONE',  #19825 ) ;
#17946=EDGE_CURVE ( 'NONE', #13870, #16962, #8714, .T. ) ;
#17950=PLANE ( 'NONE',  #10782 ) ;
#17968=ORIENTED_EDGE ( 'NONE', *, *, #13066, .T. ) ;
#17972=VECTOR ( 'NONE', #16167, 1000.000000000000000 ) ;
#17973=AXIS2_PLACEMENT_3D ( 'NONE', #227, #16550, #1736 ) ;
#17977=APPLICATION_CONTEXT ( 'automotive_design' ) ;
#17978=VECTOR ( 'NONE', #16040, 1000.000000000000000 ) ;
#17983=AXIS2_PLACEMENT_3D ( 'NONE', #16196, #6335, #1375 ) ;
#18002=EDGE_CURVE ( 'NONE', #9723, #10312, #16528, .T. ) ;
#18012=DIRECTION ( 'NONE',  ( -1.000000000000000000, 0.000000000000000000, 0.000000000000000000 ) ) ;
#18014=ORIENTED_EDGE ( 'NONE', *, *, #19607, .F. ) ;
#18016=LINE ( 'NONE', #11528, #6925 ) ;
#18019=LINE ( 'NONE', #15012, #17519 ) ;
#18020=DIRECTION ( 'NONE',  ( 1.854788578061058554E-16, 1.000000000000000000, 0.000000000000000000 ) ) ;
#18021=LINE ( 'NONE', #19642, #150 ) ;
#18034=EDGE_CURVE ( 'NONE', #3413, #14255, #4023, .T. ) ;
#18042=CIRCLE ( 'NONE', #790, 5.000000000000004441 ) ;
#18050=CARTESIAN_POINT ( 'NONE',  ( 91.21585410611801592, 56.85652257517427444, -85.46735025547123143 ) ) ;
#18057=ORIENTED_EDGE ( 'NONE', *, *, #10939, .T. ) ;
#18059=EDGE_LOOP ( 'NONE', ( #14784, #16561, #396, #15002, #2218, #5183, #10212, #20278, #4812 ) ) ;
#18070=DIRECTION ( 'NONE',  ( -1.000000000000000000, 0.000000000000000000, 0.000000000000000000 ) ) ;
#18072=DIRECTION ( 'NONE',  ( -1.000000000000000000, 0.000000000000000000, 0.000000000000000000 ) ) ;
#18078=DIRECTION ( 'NONE',  ( 1.000000000000000000, 0.000000000000000000, 0.000000000000000000 ) ) ;
#18087=ORIENTED_EDGE ( 'NONE', *, *, #1483, .T. ) ;
#18096=PRODUCT_CONTEXT ( 'NONE', #17977, 'mechanical' ) ;
#18097=DIRECTION ( 'NONE',  ( -0.000000000000000000, -0.000000000000000000, 1.000000000000000000 ) ) ;
#18101=LINE ( 'NONE', #6628, #8758 ) ;
#18102=CARTESIAN_POINT ( 'NONE',  ( 60.03793209889851568, 30.52886280891152282, 131.1729372809869005 ) ) ;
#18108=CARTESIAN_POINT ( 'NONE',  ( 20.22541975382790369, 160.1716627696692683, 61.32575462769902686 ) ) ;
#18119=EDGE_CURVE ( 'NONE', #451, #1584, #10867, .T. ) ;
#18125=CARTESIAN_POINT ( 'NONE',  ( 30.42502041961814285, 230.5765313837437418, 40.00000000000000000 ) ) ;
#18127=DIRECTION ( 'NONE',  ( 0.000000000000000000, 0.000000000000000000, 1.000000000000000000 ) ) ;
#18129=DIRECTION ( 'NONE',  ( 0.000000000000000000, 0.000000000000000000, 1.000000000000000000 ) ) ;
#18134=CARTESIAN_POINT ( 'NONE',  ( -10.76731745429009912, 56.85652257517428865, -118.3724535612433328 ) ) ;
#18138=EDGE_CURVE ( 'NONE', #763, #9302, #20403, .T. ) ;
#18139=DIRECTION ( 'NONE',  ( 0.000000000000000000, 0.000000000000000000, 1.000000000000000000 ) ) ;
#18140=EDGE_LOOP ( 'NONE', ( #2856, #9831 ) ) ;
#18144=DIRECTION ( 'NONE',  ( 0.000000000000000000, -1.000000000000000000, 0.000000000000000000 ) ) ;
#18154=( BOUNDED_CURVE ( )  B_SPLINE_CURVE ( 3, ( #8604, #4944, #11543, #18134 ),
 .UNSPECIFIED., .F., .T. ) 
 B_SPLINE_CURVE_WITH_KNOTS ( ( 4, 4 ),
 ( 4.712388980384691450, 6.283185307179586232 ),
 .UNSPECIFIED. ) 
 CURVE ( )  GEOMETRIC_REPRESENTATION_ITEM ( )  RATIONAL_B_SPLINE_CURVE ( ( 1.000000000000000000, 0.8047378541243654926, 0.8047378541243654926, 1.000000000000000000 ) ) 
 REPRESENTATION_ITEM ( '' )  );
#18157=LINE ( 'NONE', #11990, #5699 ) ;
#18163=VERTEX_POINT ( 'NONE', #9032 ) ;
#18164=VERTEX_POINT ( 'NONE', #7190 ) ;
#18167=CYLINDRICAL_SURFACE ( 'NONE', #4554, 210.7252770684331438 ) ;
#18169=VERTEX_POINT ( 'NONE', #1055 ) ;
#18174=AXIS2_PLACEMENT_3D ( 'NONE', #14006, #7161, #7380 ) ;
#18176=DIRECTION ( 'NONE',  ( 0.000000000000000000, 0.000000000000000000, 1.000000000000000000 ) ) ;
#18190=ORIENTED_EDGE ( 'NONE', *, *, #730, .F. ) ;
#18191=EDGE_LOOP ( 'NONE', ( #5388, #430, #9992, #2167, #11195, #2935, #155 ) ) ;
#18193=ADVANCED_FACE ( 'NONE', ( #14248 ), #9138, .F. ) ;
#18203=CARTESIAN_POINT ( 'NONE',  ( -10.76731745429010267, 56.32691141864442841, 46.25122601329427852 ) ) ;
#18205=FACE_OUTER_BOUND ( 'NONE', #7226, .T. ) ;
#18206=DIRECTION ( 'NONE',  ( 0.9365583756827543516, -0.000000000000000000, -0.3505116388060184329 ) ) ;
#18209=CIRCLE ( 'NONE', #16498, 125.0000000000000000 ) ;
#18210=PLANE ( 'NONE',  #15453 ) ;
#18215=CIRCLE ( 'NONE', #8542, 4.000000000000003553 ) ;
#18229=EDGE_LOOP ( 'NONE', ( #17840, #3388, #18406, #11242, #20544, #6507 ) ) ;
#18231=CARTESIAN_POINT ( 'NONE',  ( -14.71623956875115447, 48.14959005838937145, -47.59463164328435170 ) ) ;
#18236=CARTESIAN_POINT ( 'NONE',  ( 28.16023193154655502, 323.8848358243226357, 20.00000000000000355 ) ) ;
#18237=LINE ( 'NONE', #18346, #21213 ) ;
#18241=DIRECTION ( 'NONE',  ( -1.000000000000000000, 0.000000000000000000, 0.000000000000000000 ) ) ;
#18243=CARTESIAN_POINT ( 'NONE',  ( 40.42502041961814996, 180.1716627696692967, 20.00000000000000355 ) ) ;
#18247=CARTESIAN_POINT ( 'NONE',  ( -15.54750367907771746, 45.31613216062294214, 120.2864949470673110 ) ) ;
#18254=AXIS2_PLACEMENT_3D ( 'NONE', #13696, #10429, #15117 ) ;
#18264=DIRECTION ( 'NONE',  ( -1.000000000000000000, -0.000000000000000000, -0.000000000000000000 ) ) ;
#18267=ORIENTED_EDGE ( 'NONE', *, *, #17894, .T. ) ;
#18275=DIRECTION ( 'NONE',  ( -1.000000000000000000, -0.000000000000000000, -0.000000000000000000 ) ) ;
#18284=DIRECTION ( 'NONE',  ( -0.000000000000000000, 1.000000000000000000, -0.000000000000000000 ) ) ;
#18299=VERTEX_POINT ( 'NONE', #146 ) ;
#18301=ORIENTED_EDGE ( 'NONE', *, *, #4761, .T. ) ;
#18302=DIRECTION ( 'NONE',  ( 1.000000000000000000, 0.000000000000000000, 0.000000000000000000 ) ) ;
#18310=DIRECTION ( 'NONE',  ( 0.000000000000000000, 0.000000000000000000, -1.000000000000000000 ) ) ;
#18318=LINE ( 'NONE', #21144, #8167 ) ;
#18319=DIRECTION ( 'NONE',  ( 0.000000000000000000, -1.000000000000000000, 0.000000000000000000 ) ) ;
#18339=CIRCLE ( 'NONE', #7963, 49.60091809715359545 ) ;
#18341=CIRCLE ( 'NONE', #15594, 125.0000000000000000 ) ;
#18344=DIRECTION ( 'NONE',  ( 1.000000000000000000, 0.000000000000000000, -0.000000000000000000 ) ) ;
#18346=CARTESIAN_POINT ( 'NONE',  ( 91.21585410611801592, 56.85652257517428865, 94.99999999999994316 ) ) ;
#18347=FACE_OUTER_BOUND ( 'NONE', #9390, .T. ) ;
#18350=EDGE_CURVE ( 'NONE', #20033, #763, #14960, .T. ) ;
#18366=CARTESIAN_POINT ( 'NONE',  ( 91.21585410611801592, 56.85652257517428865, -94.99999999999994316 ) ) ;
#18370=VECTOR ( 'NONE', #21062, 1000.000000000000000 ) ;
#18375=CARTESIAN_POINT ( 'NONE',  ( -28.68588794268872633, 230.8848358243226073, 40.00000000000000000 ) ) ;
#18376=ORIENTED_EDGE ( 'NONE', *, *, #13546, .F. ) ;
#18379=ORIENTED_EDGE ( 'NONE', *, *, #17938, .F. ) ;
#18390=PLANE ( 'NONE',  #4122 ) ;
#18393=CARTESIAN_POINT ( 'NONE',  ( 40.42502041961814996, 170.1716627696692683, 40.00000000000000000 ) ) ;
#18396=CARTESIAN_POINT ( 'NONE',  ( -31.43424221336877622, 49.78331734519973395, 120.9832659038790865 ) ) ;
#18406=ORIENTED_EDGE ( 'NONE', *, *, #13147, .F. ) ;
#18407=CARTESIAN_POINT ( 'NONE',  ( 20.42502041961814641, 160.1716627696692683, 40.00000000000000000 ) ) ;
#18423=CARTESIAN_POINT ( 'NONE',  ( -49.57497958038185715, 160.1716627696692683, 60.00000000000000000 ) ) ;
#18425=VECTOR ( 'NONE', #4834, 1000.000000000000000 ) ;
#18426=DIRECTION ( 'NONE',  ( -1.000000000000000000, 1.854788578061058554E-16, 0.000000000000000000 ) ) ;
#18429=AXIS2_PLACEMENT_3D ( 'NONE', #3162, #3475, #25 ) ;
#18446=CARTESIAN_POINT ( 'NONE',  ( -27.08348527696885810, 46.34737952406209160, -49.57559712733488055 ) ) ;
#18447=AXIS2_PLACEMENT_3D ( 'NONE', #7008, #1957, #16667 ) ;
#18459=VERTEX_POINT ( 'NONE', #10066 ) ;
#18462=VERTEX_POINT ( 'NONE', #16689 ) ;
#18466=EDGE_CURVE ( 'NONE', #451, #7864, #6085, .T. ) ;
#18467=ORIENTED_EDGE ( 'NONE', *, *, #14867, .F. ) ;
#18468=DIRECTION ( 'NONE',  ( -0.000000000000000000, 0.000000000000000000, 1.000000000000000000 ) ) ;
#18476=EDGE_CURVE ( 'NONE', #5103, #983, #466, .T. ) ;
#18479=CARTESIAN_POINT ( 'NONE',  ( 52.60622592008805043, 30.52886280891152282, 151.0302712373927250 ) ) ;
#18490=ORIENTED_EDGE ( 'NONE', *, *, #113, .F. ) ;
#18498=PLANE ( 'NONE',  #12693 ) ;
#18502=LINE ( 'NONE', #12014, #13938 ) ;
#18508=ORIENTED_EDGE ( 'NONE', *, *, #18598, .F. ) ;
#18528=DIRECTION ( 'NONE',  ( 0.8666372666885295839, -0.4989387216749512355, 0.000000000000000000 ) ) ;
#18529=EDGE_CURVE ( 'NONE', #13714, #3284, #18502, .T. ) ;
#18530=VECTOR ( 'NONE', #15203, 1000.000000000000000 ) ;
#18537=ORIENTED_EDGE ( 'NONE', *, *, #4309, .T. ) ;
#18540=ORIENTED_EDGE ( 'NONE', *, *, #8948, .F. ) ;
#18543=ORIENTED_EDGE ( 'NONE', *, *, #10326, .F. ) ;
#18545=CARTESIAN_POINT ( 'NONE',  ( -19.19910310533017750, 45.73968925459546142, -48.68588693060413419 ) ) ;
#18550=CARTESIAN_POINT ( 'NONE',  ( 51.50493485826542184, 170.1716627696692683, -20.00000000000000355 ) ) ;
#18556=CARTESIAN_POINT ( 'NONE',  ( 115.7989814974898337, 142.5259582928263455, -40.00000000000000000 ) ) ;
#18561=CARTESIAN_POINT ( 'NONE',  ( -33.23789986170869071, 53.12371016881039054, -49.39189772945173473 ) ) ;
#18570=LINE ( 'NONE', #1834, #11806 ) ;
#18581=DIRECTION ( 'NONE',  ( -0.000000000000000000, -0.000000000000000000, -1.000000000000000000 ) ) ;
#18597=EDGE_CURVE ( 'NONE', #795, #20892, #19446, .T. ) ;
#18598=EDGE_CURVE ( 'NONE', #5454, #9142, #5410, .T. ) ;
#18600=CARTESIAN_POINT ( 'NONE',  ( 27.98965548446208373, 333.8848358243226357, -40.00000000000000000 ) ) ;
#18604=DIRECTION ( 'NONE',  ( 0.000000000000000000, -1.000000000000000000, 0.000000000000000000 ) ) ;
#18606=DIRECTION ( 'NONE',  ( -0.000000000000000000, -0.000000000000000000, -1.000000000000000000 ) ) ;
#18613=ORIENTED_EDGE ( 'NONE', *, *, #15578, .F. ) ;
#18614=LINE ( 'NONE', #3800, #12242 ) ;
#18617=CIRCLE ( 'NONE', #6509, 4.000000000000001776 ) ;
#18633=CARTESIAN_POINT ( 'NONE',  ( -32.63738144191441393, 51.69676759036851621, -120.6641474517143422 ) ) ;
#18646=CARTESIAN_POINT ( 'NONE',  ( -16.38242098736782992, 46.95008282854134052, -48.05128789156074021 ) ) ;
#18649=CARTESIAN_POINT ( 'NONE',  ( 28.16023193154655502, 323.8848358243226357, -40.00000000000000000 ) ) ;
#18650=CARTESIAN_POINT ( 'NONE',  ( 60.03793209889851568, 30.52886280891152282, 131.1729372809869005 ) ) ;
#18651=DIRECTION ( 'NONE',  ( -0.000000000000000000, -0.000000000000000000, -1.000000000000000000 ) ) ;
#18656=CARTESIAN_POINT ( 'NONE',  ( 35.96497763894179656, 191.2380552923725645, 48.74187950074039577 ) ) ;
#18658=DIRECTION ( 'NONE',  ( 0.000000000000000000, 0.000000000000000000, -1.000000000000000000 ) ) ;
#18660=FACE_OUTER_BOUND ( 'NONE', #6829, .T. ) ;
#18663=ORIENTED_EDGE ( 'NONE', *, *, #3274, .T. ) ;
#18665=DIRECTION ( 'NONE',  ( -1.232945044042657126E-32, 9.855701800883825964E-17, 1.000000000000000000 ) ) ;
#18669=VERTEX_POINT ( 'NONE', #10812 ) ;
#18684=CARTESIAN_POINT ( 'NONE',  ( -123.2946569474810019, 10.52886280891152104, -20.57735571454641388 ) ) ;
#18691=ORIENTED_EDGE ( 'NONE', *, *, #7639, .F. ) ;
#18693=ORIENTED_EDGE ( 'NONE', *, *, #5440, .T. ) ;
#18698=VERTEX_POINT ( 'NONE', #4229 ) ;
#18699=ADVANCED_FACE ( 'NONE', ( #12768 ), #4437, .F. ) ;
#18701=VERTEX_POINT ( 'NONE', #1206 ) ;
#18707=CARTESIAN_POINT ( 'NONE',  ( 91.21585410611801592, 56.85652257517428865, 94.99999999999994316 ) ) ;
#18718=ORIENTED_EDGE ( 'NONE', *, *, #15494, .T. ) ;
#18720=PLANE ( 'NONE',  #13288 ) ;
#18729=ADVANCED_FACE ( 'NONE', ( #10699 ), #9298, .F. ) ;
#18730=AXIS2_PLACEMENT_3D ( 'NONE', #940, #10861, #723 ) ;
#18742=CARTESIAN_POINT ( 'NONE',  ( 51.50493485826542184, 160.1716627696692683, -61.61851857202071159 ) ) ;
#18743=AXIS2_PLACEMENT_3D ( 'NONE', #17704, #10776, #17492 ) ;
#18751=CARTESIAN_POINT ( 'NONE',  ( 6.416697501590670427, 172.9933428177121471, 50.00000000000000000 ) ) ;
#18760=DIRECTION ( 'NONE',  ( -0.000000000000000000, -0.000000000000000000, -1.000000000000000000 ) ) ;
#18774=EDGE_LOOP ( 'NONE', ( #8428, #132, #7709, #13981 ) ) ;
#18778=ORIENTED_EDGE ( 'NONE', *, *, #6761, .F. ) ;
#18779=EDGE_CURVE ( 'NONE', #1584, #16350, #15667, .T. ) ;
#18792=AXIS2_PLACEMENT_3D ( 'NONE', #11709, #8455, #18302 ) ;
#18794=DIRECTION ( 'NONE',  ( 0.000000000000000000, 0.000000000000000000, 1.000000000000000000 ) ) ;
#18797=LINE ( 'NONE', #7433, #1186 ) ;
#18810=EDGE_CURVE ( 'NONE', #11758, #12017, #12446, .T. ) ;
#18825=EDGE_LOOP ( 'NONE', ( #12345, #3357, #19990, #1720 ) ) ;
#18827=ORIENTED_EDGE ( 'NONE', *, *, #5521, .F. ) ;
#18832=LINE ( 'NONE', #7148, #4855 ) ;
#18843=LINE ( 'NONE', #4032, #9539 ) ;
#18845=CARTESIAN_POINT ( 'NONE',  ( -33.84809828339280102, 56.08443449083164012, -120.3299889578561448 ) ) ;
#18850=VERTEX_POINT ( 'NONE', #8201 ) ;
#18852=ORIENTED_EDGE ( 'NONE', *, *, #15910, .F. ) ;
#18856=LINE ( 'NONE', #20386, #6226 ) ;
#18865=LINE ( 'NONE', #4056, #2859 ) ;
#18868=AXIS2_PLACEMENT_3D ( 'NONE', #11428, #9593, #14486 ) ;
#18885=AXIS2_PLACEMENT_3D ( 'NONE', #4520, #21276, #6029 ) ;
#18889=ORIENTED_EDGE ( 'NONE', *, *, #13069, .T. ) ;
#18893=DIRECTION ( 'NONE',  ( 0.000000000000000000, -0.000000000000000000, 1.000000000000000000 ) ) ;
#18900=VECTOR ( 'NONE', #14715, 1000.000000000000000 ) ;
#18914=ORIENTED_EDGE ( 'NONE', *, *, #19782, .T. ) ;
#18934=EDGE_LOOP ( 'NONE', ( #12647, #14651, #9144 ) ) ;
#18946=AXIS2_PLACEMENT_3D ( 'NONE', #17649, #7894, #21107 ) ;
#18947=EDGE_CURVE ( 'NONE', #8426, #16109, #12877, .T. ) ;
#18949=EDGE_CURVE ( 'NONE', #18299, #12191, #14826, .T. ) ;
#18953=LINE ( 'NONE', #13334, #5090 ) ;
#18960=EDGE_CURVE ( 'NONE', #15977, #3882, #16007, .T. ) ;
#18961=VERTEX_POINT ( 'NONE', #16092 ) ;
#18963=ORIENTED_EDGE ( 'NONE', *, *, #19394, .F. ) ;
#18965=LINE ( 'NONE', #5450, #1734 ) ;
#18968=CARTESIAN_POINT ( 'NONE',  ( 60.03793209889851568, 30.52886280891152282, -126.1729372809868863 ) ) ;
#18970=DIRECTION ( 'NONE',  ( 0.000000000000000000, 0.000000000000000000, 1.000000000000000000 ) ) ;
#18979=DIRECTION ( 'NONE',  ( -0.9283449136418786551, 0.000000000000000000, 0.3717199501173604204 ) ) ;
#18981=DIRECTION ( 'NONE',  ( 0.000000000000000000, 0.000000000000000000, 1.000000000000000000 ) ) ;
#18993=ORIENTED_EDGE ( 'NONE', *, *, #7376, .T. ) ;
#18995=EDGE_CURVE ( 'NONE', #1524, #10342, #17393, .T. ) ;
#18996=ORIENTED_EDGE ( 'NONE', *, *, #2802, .T. ) ;
#19003=PLANE ( 'NONE',  #21362 ) ;
#19005=AXIS2_PLACEMENT_3D ( 'NONE', #10634, #20496, #15638 ) ;
#19007=LINE ( 'NONE', #14158, #3593 ) ;
#19008=AXIS2_PLACEMENT_3D ( 'NONE', #14873, #18097, #9866 ) ;
#19011=CARTESIAN_POINT ( 'NONE',  ( -162.2727221670389781, 30.52886280891152282, -4.999999999999990230 ) ) ;
#19015=VECTOR ( 'NONE', #8249, 1000.000000000000000 ) ;
#19017=CIRCLE ( 'NONE', #9349, 10.00000000000000533 ) ;
#19019=CIRCLE ( 'NONE', #10373, 125.0000000000000000 ) ;
#19028=VECTOR ( 'NONE', #12731, 1000.000000000000000 ) ;
#19035=VECTOR ( 'NONE', #13703, 1000.000000000000000 ) ;
#19043=DIRECTION ( 'NONE',  ( 1.000000000000000000, 0.000000000000000000, 0.000000000000000000 ) ) ;
#19045=DIRECTION ( 'NONE',  ( 0.000000000000000000, 0.000000000000000000, 1.000000000000000000 ) ) ;
#19047=ORIENTED_EDGE ( 'NONE', *, *, #6927, .F. ) ;
#19050=VERTEX_POINT ( 'NONE', #1379 ) ;
#19059=EDGE_CURVE ( 'NONE', #16623, #7807, #6659, .T. ) ;
#19082=CARTESIAN_POINT ( 'NONE',  ( 20.42502041961813930, 230.5765313837437418, -60.00000000000000000 ) ) ;
#19083=FACE_OUTER_BOUND ( 'NONE', #18191, .T. ) ;
#19085=CIRCLE ( 'NONE', #450, 4.000000000000001776 ) ;
#19091=CARTESIAN_POINT ( 'NONE',  ( 65.85920792673738333, 160.1716627696692683, 40.00000000000000000 ) ) ;
#19092=LINE ( 'NONE', #939, #12208 ) ;
#19094=EDGE_CURVE ( 'NONE', #10871, #21097, #20150, .T. ) ;
#19095=PLANE ( 'NONE',  #13722 ) ;
#19101=CARTESIAN_POINT ( 'NONE',  ( -162.2727221670389781, 30.52886280891152282, 0.000000000000000000 ) ) ;
#19103=CYLINDRICAL_SURFACE ( 'NONE', #10584, 28.29169339157297358 ) ;
#19106=B_SPLINE_CURVE_WITH_KNOTS ( 'NONE', 3,
 ( #20062, #16611, #1801, #11835, #2320, #7163, #8900, #12155, #20374, #15311, #5658, #2111, #5758, #3931, #13786, #18633, #17139, #814, #5549, #7382, #18845, #3823 ),
 .UNSPECIFIED., .F., .F.,
 ( 4, 2, 2, 2, 2, 2, 2, 2, 2, 2, 4 ),
 ( 0.000000000000000000, 0.002281693049900210702, 0.003422539574850314101, 0.004563386099800417935, 0.006845079149700616060, 0.009126772199600815053, 0.01140846524950101318, 0.01254931177445110617, 0.01369015829940119916, 0.01597185134930136780, 0.01825354439920153643 ),
 .UNSPECIFIED. ) ;
#19111=ORIENTED_EDGE ( 'NONE', *, *, #1121, .F. ) ;
#19127=AXIS2_PLACEMENT_3D ( 'NONE', #11549, #18139, #6672 ) ;
#19156=CARTESIAN_POINT ( 'NONE',  ( 88.28695088269886071, 152.5259582928263740, -20.00000000000000355 ) ) ;
#19157=FACE_OUTER_BOUND ( 'NONE', #19342, .T. ) ;
#19163=VERTEX_POINT ( 'NONE', #3320 ) ;
#19178=DIRECTION ( 'NONE',  ( 0.000000000000000000, 0.000000000000000000, -1.000000000000000000 ) ) ;
#19182=EDGE_CURVE ( 'NONE', #2882, #15103, #8061, .T. ) ;
#19188=FACE_OUTER_BOUND ( 'NONE', #20786, .T. ) ;
#19190=DIRECTION ( 'NONE',  ( 1.000000000000000000, 1.250996701150283068E-16, -0.000000000000000000 ) ) ;
#19200=DIRECTION ( 'NONE',  ( 0.000000000000000000, 0.000000000000000000, 1.000000000000000000 ) ) ;
#19202=LINE ( 'NONE', #1051, #9209 ) ;
#19216=DIRECTION ( 'NONE',  ( 1.374938938973709817E-16, -1.000000000000000000, 0.000000000000000000 ) ) ;
#19223=DIRECTION ( 'NONE',  ( -0.000000000000000000, -0.000000000000000000, 1.000000000000000000 ) ) ;
#19228=VECTOR ( 'NONE', #865, 1000.000000000000000 ) ;
#19238=DIRECTION ( 'NONE',  ( 0.000000000000000000, 0.000000000000000000, 1.000000000000000000 ) ) ;
#19240=ORIENTED_EDGE ( 'NONE', *, *, #5382, .F. ) ;
#19243=ORIENTED_EDGE ( 'NONE', *, *, #12350, .F. ) ;
#19247=VECTOR ( 'NONE', #17260, 1000.000000000000000 ) ;
#19260=ADVANCED_FACE ( 'NONE', ( #89 ), #6656, .F. ) ;
#19266=EDGE_CURVE ( 'NONE', #9807, #13610, #10118, .T. ) ;
#19293=CYLINDRICAL_SURFACE ( 'NONE', #15252, 59.93977357075245038 ) ;
#19296=ORIENTED_EDGE ( 'NONE', *, *, #14271, .F. ) ;
#19299=LINE ( 'NONE', #14549, #2063 ) ;
#19304=CARTESIAN_POINT ( 'NONE',  ( -10.76731745429010090, 56.85652257517428865, -152.3753892284480003 ) ) ;
#19305=PLANE ( 'NONE',  #1994 ) ;
#19306=LINE ( 'NONE', #13030, #4872 ) ;
#19318=CARTESIAN_POINT ( 'NONE',  ( 65.85920792673738333, 160.1716627696692683, -20.00000000000000355 ) ) ;
#19322=LINE ( 'NONE', #2897, #399 ) ;
#19323=VECTOR ( 'NONE', #14525, 1000.000000000000000 ) ;
#19325=CARTESIAN_POINT ( 'NONE',  ( 20.42502041961813930, 230.5765313837437418, -40.00000000000000000 ) ) ;
#19329=DIRECTION ( 'NONE',  ( 1.000000000000000000, 0.000000000000000000, 0.000000000000000000 ) ) ;
#19342=EDGE_LOOP ( 'NONE', ( #20174, #20813, #19522, #20995 ) ) ;
#19343=ORIENTED_EDGE ( 'NONE', *, *, #15923, .F. ) ;
#19355=DIRECTION ( 'NONE',  ( 0.1337298367054296222, -0.9910178256594273094, 0.000000000000000000 ) ) ;
#19356=CIRCLE ( 'NONE', #15925, 5.000000000000004441 ) ;
#19360=DIRECTION ( 'NONE',  ( 0.000000000000000000, 1.000000000000000000, 0.000000000000000000 ) ) ;
#19373=CARTESIAN_POINT ( 'NONE',  ( 29.72350413846044859, 280.4463447002762564, -40.00000000000000000 ) ) ;
#19374=VECTOR ( 'NONE', #1446, 1000.000000000000000 ) ;
#19384=CARTESIAN_POINT ( 'NONE',  ( 51.50493485826542184, 141.8799693780962912, -20.00000000000000355 ) ) ;
#19385=LINE ( 'NONE', #4136, #8142 ) ;
#19394=EDGE_CURVE ( 'NONE', #13316, #10104, #20394, .T. ) ;
#19404=DIRECTION ( 'NONE',  ( 1.000000000000000000, 0.000000000000000000, -3.836511174089486666E-16 ) ) ;
#19407=CIRCLE ( 'NONE', #6272, 59.93977357075245038 ) ;
#19409=DIRECTION ( 'NONE',  ( 1.000000000000000000, 0.000000000000000000, 0.000000000000000000 ) ) ;
#19411=VECTOR ( 'NONE', #305, 1000.000000000000000 ) ;
#19412=LINE ( 'NONE', #9245, #3687 ) ;
#19415=DIRECTION ( 'NONE',  ( 1.000000000000000000, 1.250996701150283068E-16, -0.000000000000000000 ) ) ;
#19420=ORIENTED_EDGE ( 'NONE', *, *, #1523, .F. ) ;
#19424=ORIENTED_EDGE ( 'NONE', *, *, #9858, .F. ) ;
#19428=DIRECTION ( 'NONE',  ( 0.000000000000000000, 0.000000000000000000, 1.000000000000000000 ) ) ;
#19429=CARTESIAN_POINT ( 'NONE',  ( 60.03793209889851568, 30.52886280891152282, -131.1729372809869005 ) ) ;
#19436=AXIS2_PLACEMENT_3D ( 'NONE', #18236, #13490, #8388 ) ;
#19437=LINE ( 'NONE', #4620, #21142 ) ;
#19438=FACE_BOUND ( 'NONE', #7064, .T. ) ;
#19446=CIRCLE ( 'NONE', #117, 4.000000000000003553 ) ;
#19453=VERTEX_POINT ( 'NONE', #11073 ) ;
#19463=ADVANCED_FACE ( 'NONE', ( #12608 ), #6204, .F. ) ;
#19464=PLANE ( 'NONE',  #9914 ) ;
#19469=ORIENTED_EDGE ( 'NONE', *, *, #2364, .T. ) ;
#19477=DIRECTION ( 'NONE',  ( -1.000000000000000000, 0.000000000000000000, 0.000000000000000000 ) ) ;
#19479=EDGE_CURVE ( 'NONE', #2963, #12191, #17574, .T. ) ;
#19483=CARTESIAN_POINT ( 'NONE',  ( 35.96497763894178945, 230.5765313837437418, -60.00000000000000000 ) ) ;
#19490=EDGE_CURVE ( 'NONE', #2298, #2858, #3242, .T. ) ;
#19494=CIRCLE ( 'NONE', #18792, 10.00000000000000178 ) ;
#19502=DIRECTION ( 'NONE',  ( -0.000000000000000000, -0.000000000000000000, -1.000000000000000000 ) ) ;
#19511=CARTESIAN_POINT ( 'NONE',  ( -27.55128289072937875, 46.57285964785339161, 49.58849804005138395 ) ) ;
#19512=FACE_BOUND ( 'NONE', #1143, .T. ) ;
#19514=DIRECTION ( 'NONE',  ( 0.000000000000000000, -1.000000000000000000, 0.000000000000000000 ) ) ;
#19516=CARTESIAN_POINT ( 'NONE',  ( 51.98438129372387806, 30.52886280891151216, 94.99999999999994316 ) ) ;
#19520=CARTESIAN_POINT ( 'NONE',  ( 20.42502041961806825, 281.1055109169419666, 20.00000000000000355 ) ) ;
#19522=ORIENTED_EDGE ( 'NONE', *, *, #5783, .F. ) ;
#19528=EDGE_CURVE ( 'NONE', #20892, #12520, #4378, .T. ) ;
#19535=DIRECTION ( 'NONE',  ( 0.000000000000000000, 0.000000000000000000, 1.000000000000000000 ) ) ;
#19541=FACE_BOUND ( 'NONE', #1525, .T. ) ;
#19552=ORIENTED_EDGE ( 'NONE', *, *, #15044, .T. ) ;
#19571=VERTEX_POINT ( 'NONE', #9345 ) ;
#19584=CARTESIAN_POINT ( 'NONE',  ( 40.42502041961814996, 170.1716627696692683, 20.00000000000000355 ) ) ;
#19586=AXIS2_PLACEMENT_3D ( 'NONE', #12150, #18426, #10197 ) ;
#19593=DIRECTION ( 'NONE',  ( 0.000000000000000000, 0.000000000000000000, 1.000000000000000000 ) ) ;
#19606=DIRECTION ( 'NONE',  ( 0.000000000000000000, -1.000000000000000000, 0.000000000000000000 ) ) ;
#19607=EDGE_CURVE ( 'NONE', #19679, #15845, #19092, .T. ) ;
#19609=CARTESIAN_POINT ( 'NONE',  ( 20.42502041961813575, 271.1055109169419666, 40.00000000000000000 ) ) ;
#19613=FACE_OUTER_BOUND ( 'NONE', #20069, .T. ) ;
#19615=CARTESIAN_POINT ( 'NONE',  ( -11.91936617617171734, 51.80349839367686826, 46.68171932492850829 ) ) ;
#19617=CARTESIAN_POINT ( 'NONE',  ( -28.68588794268874054, 271.1055109169419666, -40.00000000000000000 ) ) ;
#19622=LINE ( 'NONE', #68, #17158 ) ;
#19642=CARTESIAN_POINT ( 'NONE',  ( 91.21585410611801592, 56.85652257517428865, 94.99999999999994316 ) ) ;
#19643=DIRECTION ( 'NONE',  ( 1.250996701150283068E-16, -1.000000000000000000, 0.000000000000000000 ) ) ;
#19644=VECTOR ( 'NONE', #5149, 1000.000000000000000 ) ;
#19655=VERTEX_POINT ( 'NONE', #4276 ) ;
#19677=VERTEX_POINT ( 'NONE', #14767 ) ;
#19679=VERTEX_POINT ( 'NONE', #17884 ) ;
#19683=DIRECTION ( 'NONE',  ( 0.000000000000000000, 0.000000000000000000, -1.000000000000000000 ) ) ;
#19708=CIRCLE ( 'NONE', #4853, 28.29169339157297358 ) ;
#19710=ORIENTED_EDGE ( 'NONE', *, *, #7363, .T. ) ;
#19711=CARTESIAN_POINT ( 'NONE',  ( -28.68588794268873343, 47.23886018424757083, 49.60091809715359545 ) ) ;
#19720=DIRECTION ( 'NONE',  ( 0.000000000000000000, 1.000000000000000000, 0.000000000000000000 ) ) ;
#19721=LINE ( 'NONE', #20384, #16368 ) ;
#19723=CARTESIAN_POINT ( 'NONE',  ( -24.85377105065298764, 45.59741950151473588, 49.45332593944714716 ) ) ;
#19724=DIRECTION ( 'NONE',  ( 0.000000000000000000, 1.000000000000000000, 9.855701800883825964E-17 ) ) ;
#19734=LINE ( 'NONE', #393, #12329 ) ;
#19738=ORIENTED_EDGE ( 'NONE', *, *, #11264, .F. ) ;
#19741=ORIENTED_EDGE ( 'NONE', *, *, #4546, .T. ) ;
#19750=DIRECTION ( 'NONE',  ( -0.000000000000000000, -0.000000000000000000, -1.000000000000000000 ) ) ;
#19753=LINE ( 'NONE', #1175, #8712 ) ;
#19765=ORIENTED_EDGE ( 'NONE', *, *, #21337, .T. ) ;
#19782=EDGE_CURVE ( 'NONE', #19453, #9142, #3187, .T. ) ;
#19785=ADVANCED_FACE ( 'NONE', ( #6519 ), #1566, .F. ) ;
#19787=CARTESIAN_POINT ( 'NONE',  ( 30.42502041961813575, 271.1055109169419097, -40.00000000000000000 ) ) ;
#19788=ORIENTED_EDGE ( 'NONE', *, *, #5960, .F. ) ;
#19796=ADVANCED_FACE ( 'NONE', ( #8248 ), #1792, .F. ) ;
#19799=ORIENTED_EDGE ( 'NONE', *, *, #11993, .F. ) ;
#19804=AXIS2_PLACEMENT_3D ( 'NONE', #5040, #8387, #18344 ) ;
#19806=EDGE_CURVE ( 'NONE', #5497, #451, #836, .T. ) ;
#19817=EDGE_CURVE ( 'NONE', #17482, #12966, #18101, .T. ) ;
#19825=AXIS2_PLACEMENT_3D ( 'NONE', #3140, #14509, #9722 ) ;
#19827=VERTEX_POINT ( 'NONE', #19838 ) ;
#19831=DIRECTION ( 'NONE',  ( -1.000000000000000000, 0.000000000000000000, 0.000000000000000000 ) ) ;
#19836=CARTESIAN_POINT ( 'NONE',  ( -10.80396482869975472, 55.79733835392248409, 46.26547175773355747 ) ) ;
#19837=DIRECTION ( 'NONE',  ( 1.000000000000000000, 0.000000000000000000, 0.000000000000000000 ) ) ;
#19838=CARTESIAN_POINT ( 'NONE',  ( 60.69669829156632090, 56.85652257517428865, 94.99999999999994316 ) ) ;
#19845=LINE ( 'NONE', #8256, #18530 ) ;
#19853=VERTEX_POINT ( 'NONE', #11614 ) ;
#19858=CARTESIAN_POINT ( 'NONE',  ( -15.10870380797810952, 47.82216028940542429, -47.70846432324336917 ) ) ;
#19859=ADVANCED_FACE ( 'NONE', ( #18205 ), #6740, .F. ) ;
#19864=FACE_OUTER_BOUND ( 'NONE', #14044, .T. ) ;
#19868=DIRECTION ( 'NONE',  ( 1.374938938973709817E-16, -1.000000000000000000, 0.000000000000000000 ) ) ;
#19874=ADVANCED_FACE ( 'NONE', ( #19913 ), #8110, .T. ) ;
#19883=ADVANCED_FACE ( 'NONE', ( #5094 ), #1539, .T. ) ;
#19889=CARTESIAN_POINT ( 'NONE',  ( 91.21585410611801592, 31.85652257517428865, -40.00000000000000000 ) ) ;
#19895=LINE ( 'NONE', #18375, #154 ) ;
#19898=ORIENTED_EDGE ( 'NONE', *, *, #17107, .F. ) ;
#19899=ORIENTED_EDGE ( 'NONE', *, *, #16104, .T. ) ;
#19903=CARTESIAN_POINT ( 'NONE',  ( 292.4526463419396691, 308.2087638784415162, 40.00000000000000000 ) ) ;
#19913=FACE_OUTER_BOUND ( 'NONE', #16510, .T. ) ;
#19915=AXIS2_PLACEMENT_3D ( 'NONE', #647, #9162, #14164 ) ;
#19917=CARTESIAN_POINT ( 'NONE',  ( 91.21585410611801592, 56.85652257517428865, 94.99999999999994316 ) ) ;
#19925=ORIENTED_EDGE ( 'NONE', *, *, #16291, .F. ) ;
#19928=EDGE_CURVE ( 'NONE', #18459, #15711, #11870, .T. ) ;
#19932=DIRECTION ( 'NONE',  ( 0.000000000000000000, -0.000000000000000000, -1.000000000000000000 ) ) ;
#19943=CARTESIAN_POINT ( 'NONE',  ( 35.96497763894178945, 230.5765313837437418, 40.00000000000000000 ) ) ;
#19944=DIRECTION ( 'NONE',  ( -1.232945044042657126E-32, 9.855701800883825964E-17, -1.000000000000000000 ) ) ;
#19953=CIRCLE ( 'NONE', #9224, 22.72497359561857877 ) ;
#19966=ORIENTED_EDGE ( 'NONE', *, *, #2184, .F. ) ;
#19968=CARTESIAN_POINT ( 'NONE',  ( -17.74224102826533311, 46.24521970153912065, -48.38107137947394421 ) ) ;
#19980=CARTESIAN_POINT ( 'NONE',  ( -32.69826294449585191, 51.81229826077375833, -49.43888307834195928 ) ) ;
#19983=DIRECTION ( 'NONE',  ( -0.000000000000000000, -0.000000000000000000, -1.000000000000000000 ) ) ;
#19987=EDGE_CURVE ( 'NONE', #7807, #4231, #4987, .T. ) ;
#19990=ORIENTED_EDGE ( 'NONE', *, *, #6980, .T. ) ;
#20003=AXIS2_PLACEMENT_3D ( 'NONE', #8571, #15194, #11720 ) ;
#20004=EDGE_CURVE ( 'NONE', #13368, #20443, #15681, .T. ) ;
#20013=VECTOR ( 'NONE', #17905, 1000.000000000000114 ) ;
#20015=CARTESIAN_POINT ( 'NONE',  ( 65.85920792673738333, 160.1716627696692683, 40.00000000000000000 ) ) ;
#20016=ORIENTED_EDGE ( 'NONE', *, *, #14468, .T. ) ;
#20027=CARTESIAN_POINT ( 'NONE',  ( -24.92302309252174197, 45.61007917770206888, 122.4907538390011439 ) ) ;
#20033=VERTEX_POINT ( 'NONE', #2284 ) ;
#20036=ORIENTED_EDGE ( 'NONE', *, *, #13730, .T. ) ;
#20038=ORIENTED_EDGE ( 'NONE', *, *, #8287, .F. ) ;
#20041=DIRECTION ( 'NONE',  ( -0.000000000000000000, 1.000000000000000000, -0.000000000000000000 ) ) ;
#20045=VECTOR ( 'NONE', #7496, 1000.000000000000000 ) ;
#20048=CIRCLE ( 'NONE', #21079, 125.0000000000000000 ) ;
#20049=DIRECTION ( 'NONE',  ( 0.000000000000000000, 0.000000000000000000, 1.000000000000000000 ) ) ;
#20054=CARTESIAN_POINT ( 'NONE',  ( 52.60622592008805043, 10.52886280891152104, -151.0302712373927250 ) ) ;
#20057=PLANE ( 'NONE',  #19586 ) ;
#20058=LINE ( 'NONE', #3405, #16289 ) ;
#20062=CARTESIAN_POINT ( 'NONE',  ( -22.30770786884144741, 45.31613216062291372, -122.9933582338429687 ) ) ;
#20063=EDGE_CURVE ( 'NONE', #534, #1580, #7342, .T. ) ;
#20069=EDGE_LOOP ( 'NONE', ( #20728, #10070, #8378, #3457 ) ) ;
#20073=ORIENTED_EDGE ( 'NONE', *, *, #7215, .T. ) ;
#20076=ORIENTED_EDGE ( 'NONE', *, *, #10354, .F. ) ;
#20078=CARTESIAN_POINT ( 'NONE',  ( -20.71406170972610639, 45.37974668544075740, -48.96689081729963533 ) ) ;
#20079=VECTOR ( 'NONE', #3739, 1000.000000000000000 ) ;
#20081=VECTOR ( 'NONE', #3271, 1000.000000000000000 ) ;
#20090=DIRECTION ( 'NONE',  ( -0.000000000000000000, -0.000000000000000000, 1.000000000000000000 ) ) ;
#20094=ORIENTED_EDGE ( 'NONE', *, *, #5960, .T. ) ;
#20107=FACE_OUTER_BOUND ( 'NONE', #11137, .T. ) ;
#20119=ORIENTED_EDGE ( 'NONE', *, *, #1382, .T. ) ;
#20120=VERTEX_POINT ( 'NONE', #7129 ) ;
#20125=ORIENTED_EDGE ( 'NONE', *, *, #7023, .F. ) ;
#20127=ORIENTED_EDGE ( 'NONE', *, *, #5457, .F. ) ;
#20132=CARTESIAN_POINT ( 'NONE',  ( 292.4526463419396691, 308.2087638784415162, -40.00000000000000000 ) ) ;
#20134=DIRECTION ( 'NONE',  ( 1.000000000000000000, 0.000000000000000000, 0.000000000000000000 ) ) ;
#20135=AXIS2_PLACEMENT_3D ( 'NONE', #6205, #4693, #6313 ) ;
#20146=ADVANCED_FACE ( 'NONE', ( #13755 ), #12231, .F. ) ;
#20150=CIRCLE ( 'NONE', #18743, 220.7252770684331438 ) ;
#20153=CARTESIAN_POINT ( 'NONE',  ( 65.85920792673738333, 160.1716627696692683, -20.00000000000000355 ) ) ;
#20158=CARTESIAN_POINT ( 'NONE',  ( 0.000000000000000000, 31.85652257517428865, 0.000000000000000000 ) ) ;
#20165=VECTOR ( 'NONE', #7569, 1000.000000000000000 ) ;
#20169=AXIS2_PLACEMENT_3D ( 'NONE', #7506, #7400, #17679 ) ;
#20174=ORIENTED_EDGE ( 'NONE', *, *, #2670, .T. ) ;
#20176=ORIENTED_EDGE ( 'NONE', *, *, #9538, .F. ) ;
#20180=ORIENTED_EDGE ( 'NONE', *, *, #4332, .T. ) ;
#20185=CARTESIAN_POINT ( 'NONE',  ( -162.2727221670389781, 10.52886280891152104, -20.57735571454641033 ) ) ;
#20188=DIRECTION ( 'NONE',  ( -9.855701800883827197E-17, 1.000000000000000000, -0.000000000000000000 ) ) ;
#20192=CARTESIAN_POINT ( 'NONE',  ( -32.89690641512254388, 52.24437994842455879, -49.42213772442809727 ) ) ;
#20196=ORIENTED_EDGE ( 'NONE', *, *, #3336, .F. ) ;
#20197=CARTESIAN_POINT ( 'NONE',  ( 20.42502041961814641, 160.1716627696692683, 40.00000000000000000 ) ) ;
#20222=ORIENTED_EDGE ( 'NONE', *, *, #1749, .F. ) ;
#20232=DIRECTION ( 'NONE',  ( 0.9997392892938121722, 0.02283316540262222971, 0.000000000000000000 ) ) ;
#20236=CARTESIAN_POINT ( 'NONE',  ( -22.30770786884143675, 45.31613216062291372, 122.9933582338429687 ) ) ;
#20238=DIRECTION ( 'NONE',  ( 0.000000000000000000, -1.000000000000000000, 0.000000000000000000 ) ) ;
#20245=ORIENTED_EDGE ( 'NONE', *, *, #12935, .T. ) ;
#20247=ORIENTED_EDGE ( 'NONE', *, *, #16571, .T. ) ;
#20255=EDGE_CURVE ( 'NONE', #10342, #15817, #14332, .T. ) ;
#20265=DIRECTION ( 'NONE',  ( -0.000000000000000000, -0.000000000000000000, 1.000000000000000000 ) ) ;
#20269=AXIS2_PLACEMENT_3D ( 'NONE', #6239, #16210, #16003 ) ;
#20276=ORIENTED_EDGE ( 'NONE', *, *, #7639, .T. ) ;
#20278=ORIENTED_EDGE ( 'NONE', *, *, #17163, .F. ) ;
#20281=LINE ( 'NONE', #9121, #20045 ) ;
#20284=ORIENTED_EDGE ( 'NONE', *, *, #1295, .T. ) ;
#20286=CARTESIAN_POINT ( 'NONE',  ( -23.04382792501472821, 45.33667810281676935, -49.27968317789310504 ) ) ;
#20302=EDGE_CURVE ( 'NONE', #16730, #18163, #5806, .T. ) ;
#20311=ORIENTED_EDGE ( 'NONE', *, *, #4063, .F. ) ;
#20312=CARTESIAN_POINT ( 'NONE',  ( -18.68588794268873698, 323.8848358243226357, 20.00000000000000355 ) ) ;
#20314=CARTESIAN_POINT ( 'NONE',  ( 69.55160839065807465, 152.8169032537915086, -64.80145223029052204 ) ) ;
#20323=ADVANCED_FACE ( 'NONE', ( #10885, #7643, #5595 ), #7422, .T. ) ;
#20326=EDGE_CURVE ( 'NONE', #19827, #15737, #18021, .T. ) ;
#20327=EDGE_LOOP ( 'NONE', ( #8530, #2726, #17903, #443 ) ) ;
#20345=CARTESIAN_POINT ( 'NONE',  ( 105.7989814974898479, 152.5259582928263740, 40.00000000000000000 ) ) ;
#20349=EDGE_LOOP ( 'NONE', ( #3440, #17453, #7142, #6142, #15028, #15659 ) ) ;
#20353=ORIENTED_EDGE ( 'NONE', *, *, #1303, .T. ) ;
#20357=VECTOR ( 'NONE', #17857, 1000.000000000000000 ) ;
#20366=DIRECTION ( 'NONE',  ( -0.000000000000000000, 1.000000000000000000, -0.000000000000000000 ) ) ;
#20374=CARTESIAN_POINT ( 'NONE',  ( -28.05147542941067229, 46.81912526956768517, -121.8134868412888494 ) ) ;
#20383=DIRECTION ( 'NONE',  ( -0.000000000000000000, -0.000000000000000000, -1.000000000000000000 ) ) ;
#20384=CARTESIAN_POINT ( 'NONE',  ( -123.2946569474810161, 30.52886280891152282, 20.57735571454641388 ) ) ;
#20385=CARTESIAN_POINT ( 'NONE',  ( -10.76731745429010090, 56.85652257517428865, 46.25122601329427141 ) ) ;
#20386=CARTESIAN_POINT ( 'NONE',  ( 30.42502041961814996, 170.1716627696692683, 20.00000000000000355 ) ) ;
#20394=LINE ( 'NONE', #17053, #17403 ) ;
#20403=LINE ( 'NONE', #12395, #15102 ) ;
#20407=EDGE_LOOP ( 'NONE', ( #6856, #8800, #10112, #11140 ) ) ;
#20408=CIRCLE ( 'NONE', #12062, 10.00000000000000178 ) ;
#20409=CARTESIAN_POINT ( 'NONE',  ( 6.416697501590670427, 172.9933428177121471, 50.00000000000000000 ) ) ;
#20411=EDGE_CURVE ( 'NONE', #2296, #1002, #19753, .T. ) ;
#20420=DIRECTION ( 'NONE',  ( -0.000000000000000000, 1.000000000000000000, -0.000000000000000000 ) ) ;
#20422=EDGE_CURVE ( 'NONE', #8699, #19163, #14478, .T. ) ;
#20429=VECTOR ( 'NONE', #3464, 1000.000000000000000 ) ;
#20440=ORIENTED_EDGE ( 'NONE', *, *, #12390, .T. ) ;
#20443=VERTEX_POINT ( 'NONE', #14693 ) ;
#20450=ADVANCED_FACE ( 'NONE', ( #19541, #2792, #11420 ), #9587, .F. ) ;
#20463=ORIENTED_EDGE ( 'NONE', *, *, #3021, .T. ) ;
#20464=CARTESIAN_POINT ( 'NONE',  ( -49.57497958038186425, 230.5765313837437418, 49.99999999999999289 ) ) ;
#20466=ORIENTED_EDGE ( 'NONE', *, *, #730, .T. ) ;
#20482=DIRECTION ( 'NONE',  ( 0.9999562017632421806, 0.000000000000000000, 0.009359196291876339252 ) ) ;
#20484=DIRECTION ( 'NONE',  ( -0.000000000000000000, -0.000000000000000000, 1.000000000000000000 ) ) ;
#20492=ORIENTED_EDGE ( 'NONE', *, *, #13291, .T. ) ;
#20495=PLANE ( 'NONE',  #15344 ) ;
#20496=DIRECTION ( 'NONE',  ( 0.000000000000000000, 1.000000000000000000, 0.000000000000000000 ) ) ;
#20499=ORIENTED_EDGE ( 'NONE', *, *, #1392, .F. ) ;
#20518=VECTOR ( 'NONE', #7710, 999.9999999999998863 ) ;
#20529=DIRECTION ( 'NONE',  ( -9.855701800883827197E-17, 1.000000000000000000, 9.855701800883827197E-17 ) ) ;
#20534=CARTESIAN_POINT ( 'NONE',  ( 60.03793209889851568, 30.52886280891152282, 126.1729372809868863 ) ) ;
#20539=CARTESIAN_POINT ( 'NONE',  ( -49.57497958038185715, 160.1716627696692683, 60.00000000000000000 ) ) ;
#20543=ADVANCED_FACE ( 'NONE', ( #5041 ), #11641, .F. ) ;
#20544=ORIENTED_EDGE ( 'NONE', *, *, #5382, .T. ) ;
#20546=ORIENTED_EDGE ( 'NONE', *, *, #16856, .F. ) ;
#20560=CARTESIAN_POINT ( 'NONE',  ( 51.98438129372387806, 56.85652257517428865, -117.7249735956185219 ) ) ;
#20562=CIRCLE ( 'NONE', #15696, 43.46661168214937732 ) ;
#20568=ORIENTED_EDGE ( 'NONE', *, *, #18598, .T. ) ;
#20588=FACE_OUTER_BOUND ( 'NONE', #7779, .T. ) ;
#20591=ORIENTED_EDGE ( 'NONE', *, *, #4309, .F. ) ;
#20597=DIRECTION ( 'NONE',  ( -0.000000000000000000, -1.000000000000000000, -0.000000000000000000 ) ) ;
#20599=ORIENTED_EDGE ( 'NONE', *, *, #1256, .F. ) ;
#20605=CARTESIAN_POINT ( 'NONE',  ( 10.41669750159067220, 217.7548513357008630, 45.00000000000000000 ) ) ;
#20607=VECTOR ( 'NONE', #10729, 1000.000000000000000 ) ;
#20610=LINE ( 'NONE', #18656, #4523 ) ;
#20616=FACE_OUTER_BOUND ( 'NONE', #11554, .T. ) ;
#20618=ORIENTED_EDGE ( 'NONE', *, *, #13021, .F. ) ;
#20623=ORIENTED_EDGE ( 'NONE', *, *, #9208, .F. ) ;
#20632=DIRECTION ( 'NONE',  ( -0.000000000000000000, 0.000000000000000000, 1.000000000000000000 ) ) ;
#20636=LINE ( 'NONE', #19011, #14592 ) ;
#20639=VECTOR ( 'NONE', #13194, 1000.000000000000000 ) ;
#20640=CARTESIAN_POINT ( 'NONE',  ( 115.7989814974898195, 160.1716627696691830, -20.00000000000000355 ) ) ;
#20644=EDGE_CURVE ( 'NONE', #1316, #13, #6871, .T. ) ;
#20649=ORIENTED_EDGE ( 'NONE', *, *, #14352, .T. ) ;
#20650=ORIENTED_EDGE ( 'NONE', *, *, #6035, .F. ) ;
#20652=DIRECTION ( 'NONE',  ( 1.000000000000000000, 0.000000000000000000, 0.000000000000000000 ) ) ;
#20653=ORIENTED_EDGE ( 'NONE', *, *, #10446, .F. ) ;
#20664=LINE ( 'NONE', #4227, #11655 ) ;
#20670=ORIENTED_EDGE ( 'NONE', *, *, #7618, .T. ) ;
#20672=VERTEX_POINT ( 'NONE', #5355 ) ;
#20673=ORIENTED_EDGE ( 'NONE', *, *, #3842, .F. ) ;
#20679=CARTESIAN_POINT ( 'NONE',  ( 115.7989814974898195, 160.1716627696692683, 40.00000000000000000 ) ) ;
#20685=AXIS2_PLACEMENT_3D ( 'NONE', #12621, #3090, #8046 ) ;
#20689=SHAPE_REPRESENTATION_RELATIONSHIP ( 'NONE' , 'NONE' ,  #21199, #7644 ) ;
#20694=CARTESIAN_POINT ( 'NONE',  ( -123.2946569474810161, 30.52886280891152282, 20.57735571454641388 ) ) ;
#20699=AXIS2_PLACEMENT_3D ( 'NONE', #6202, #9023, #5778 ) ;
#20702=VERTEX_POINT ( 'NONE', #6657 ) ;
#20706=AXIS2_PLACEMENT_3D ( 'NONE', #1562, #11179, #17673 ) ;
#20707=CARTESIAN_POINT ( 'NONE',  ( -28.68588794268872633, 230.8848358243226073, 0.000000000000000000 ) ) ;
#20717=CARTESIAN_POINT ( 'NONE',  ( -28.68588794268874054, 333.8848358243226357, 40.00000000000000000 ) ) ;
#20724=DIRECTION ( 'NONE',  ( 0.000000000000000000, -1.000000000000000000, 0.000000000000000000 ) ) ;
#20728=ORIENTED_EDGE ( 'NONE', *, *, #15717, .F. ) ;
#20733=ADVANCED_FACE ( 'NONE', ( #1820 ), #6978, .F. ) ;
#20740=ADVANCED_FACE ( 'NONE', ( #19864 ), #16632, .F. ) ;
#20742=CARTESIAN_POINT ( 'NONE',  ( 115.7989814974898337, 152.5259582928263740, -20.00000000000000355 ) ) ;
#20746=CARTESIAN_POINT ( 'NONE',  ( 91.21585410611801592, 56.85652257517428865, -94.99999999999994316 ) ) ;
#20749=ADVANCED_FACE ( 'NONE', ( #16843 ), #13385, .F. ) ;
#20773=VECTOR ( 'NONE', #4135, 1000.000000000000114 ) ;
#20785=EDGE_LOOP ( 'NONE', ( #8055, #21124, #4174 ) ) ;
#20786=EDGE_LOOP ( 'NONE', ( #13792, #4296, #2462, #20311 ) ) ;
#20787=ORIENTED_EDGE ( 'NONE', *, *, #19806, .F. ) ;
#20789=VECTOR ( 'NONE', #20652, 1000.000000000000000 ) ;
#20811=ORIENTED_EDGE ( 'NONE', *, *, #5051, .F. ) ;
#20813=ORIENTED_EDGE ( 'NONE', *, *, #12784, .F. ) ;
#20819=LINE ( 'NONE', #4899, #17972 ) ;
#20821=VECTOR ( 'NONE', #861, 1000.000000000000000 ) ;
#20827=CARTESIAN_POINT ( 'NONE',  ( -123.2946569474810019, -343.0245277843623057, -20.57735571454641388 ) ) ;
#20828=DIRECTION ( 'NONE',  ( -0.000000000000000000, -0.000000000000000000, 1.000000000000000000 ) ) ;
#20830=DIRECTION ( 'NONE',  ( 1.000000000000000000, 1.250996701150283068E-16, -0.000000000000000000 ) ) ;
#20847=VECTOR ( 'NONE', #3137, 1000.000000000000114 ) ;
#20848=ORIENTED_EDGE ( 'NONE', *, *, #3225, .F. ) ;
#20863=ADVANCED_FACE ( 'NONE', ( #15541 ), #1046, .F. ) ;
#20883=DIRECTION ( 'NONE',  ( 0.1337298367054296222, -0.9910178256594273094, 0.000000000000000000 ) ) ;
#20892=VERTEX_POINT ( 'NONE', #12502 ) ;
#20896=DIRECTION ( 'NONE',  ( -0.000000000000000000, -0.000000000000000000, 1.000000000000000000 ) ) ;
#20902=DIRECTION ( 'NONE',  ( 1.000000000000000000, 0.000000000000000000, 0.000000000000000000 ) ) ;
#20906=CARTESIAN_POINT ( 'NONE',  ( -162.2727221670389781, 30.52886280891152282, 0.000000000000000000 ) ) ;
#20918=CARTESIAN_POINT ( 'NONE',  ( -74.06037022053952512, 10.52886280891152104, 40.00000000000000000 ) ) ;
#20928=PLANE ( 'NONE',  #10943 ) ;
#20930=CARTESIAN_POINT ( 'NONE',  ( -28.68588794268872633, 333.8848358243226357, 0.000000000000000000 ) ) ;
#20942=CARTESIAN_POINT ( 'NONE',  ( 20.42502041961806825, 281.1055109169419666, 40.00000000000000000 ) ) ;
#20946=ORIENTED_EDGE ( 'NONE', *, *, #15237, .T. ) ;
#20949=ORIENTED_EDGE ( 'NONE', *, *, #18466, .T. ) ;
#20951=LINE ( 'NONE', #21055, #13847 ) ;
#20952=EDGE_CURVE ( 'NONE', #8903, #13483, #18865, .T. ) ;
#20955=PLANE ( 'NONE',  #9955 ) ;
#20958=PLANE ( 'NONE',  #11529 ) ;
#20973=ORIENTED_EDGE ( 'NONE', *, *, #10803, .T. ) ;
#20974=ORIENTED_EDGE ( 'NONE', *, *, #8688, .T. ) ;
#20976=DIRECTION ( 'NONE',  ( 0.000000000000000000, 0.000000000000000000, -1.000000000000000000 ) ) ;
#20986=CARTESIAN_POINT ( 'NONE',  ( 30.42502041961813575, 271.1055109169419097, 40.00000000000000000 ) ) ;
#20988=EDGE_CURVE ( 'NONE', #15711, #18459, #13223, .T. ) ;
#20990=EDGE_CURVE ( 'NONE', #258, #13483, #16392, .T. ) ;
#20993=EDGE_LOOP ( 'NONE', ( #8528, #13125 ) ) ;
#20995=ORIENTED_EDGE ( 'NONE', *, *, #2551, .T. ) ;
#20996=ORIENTED_EDGE ( 'NONE', *, *, #9021, .F. ) ;
#21000=DIRECTION ( 'NONE',  ( 0.000000000000000000, 0.000000000000000000, -1.000000000000000000 ) ) ;
#21008=CARTESIAN_POINT ( 'NONE',  ( 91.21585410611801592, 31.85652257517428865, 40.00000000000000000 ) ) ;
#21023=AXIS2_PLACEMENT_3D ( 'NONE', #5253, #11852, #299 ) ;
#21029=PLANE ( 'NONE',  #2432 ) ;
#21034=DIRECTION ( 'NONE',  ( 0.000000000000000000, 1.000000000000000000, 0.000000000000000000 ) ) ;
#21038=EDGE_CURVE ( 'NONE', #3421, #18163, #8369, .T. ) ;
#21055=CARTESIAN_POINT ( 'NONE',  ( 65.85920792673738333, 170.1716627696692683, 40.00000000000000000 ) ) ;
#21061=DIRECTION ( 'NONE',  ( 0.9283449136418786551, 0.000000000000000000, -0.3717199501173604204 ) ) ;
#21062=DIRECTION ( 'NONE',  ( 1.000000000000000000, 1.250996701150283068E-16, -0.000000000000000000 ) ) ;
#21073=LINE ( 'NONE', #15897, #2889 ) ;
#21074=EDGE_LOOP ( 'NONE', ( #11519, #2807, #15270, #14709, #1242, #13207 ) ) ;
#21079=AXIS2_PLACEMENT_3D ( 'NONE', #4687, #16279, #11282 ) ;
#21080=EDGE_CURVE ( 'NONE', #20702, #20033, #17680, .T. ) ;
#21088=AXIS2_PLACEMENT_3D ( 'NONE', #17148, #2539, #18970 ) ;
#21097=VERTEX_POINT ( 'NONE', #12712 ) ;
#21107=DIRECTION ( 'NONE',  ( 0.000000000000000000, 0.000000000000000000, -1.000000000000000000 ) ) ;
#21117=ADVANCED_FACE ( 'NONE', ( #1151 ), #6412, .T. ) ;
#21123=ADVANCED_FACE ( 'NONE', ( #14666 ), #2873, .F. ) ;
#21124=ORIENTED_EDGE ( 'NONE', *, *, #9021, .T. ) ;
#21125=CARTESIAN_POINT ( 'NONE',  ( -18.68588794268873698, 281.1055109169419666, -20.00000000000000355 ) ) ;
#21127=FACE_OUTER_BOUND ( 'NONE', #3095, .T. ) ;
#21132=ORIENTED_EDGE ( 'NONE', *, *, #21391, .F. ) ;
#21135=DIRECTION ( 'NONE',  ( -1.000000000000000000, 0.000000000000000000, 0.000000000000000000 ) ) ;
#21138=CARTESIAN_POINT ( 'NONE',  ( -23.82219669152593156, 45.40396441825297558, 49.36459573994701344 ) ) ;
#21141=CARTESIAN_POINT ( 'NONE',  ( -162.2727221670389781, 10.52886280891152104, 0.000000000000000000 ) ) ;
#21142=VECTOR ( 'NONE', #17814, 1000.000000000000114 ) ;
#21144=CARTESIAN_POINT ( 'NONE',  ( 60.69669829156632090, 56.85652257517428865, -94.99999999999994316 ) ) ;
#21153=EDGE_LOOP ( 'NONE', ( #18996, #20127, #15661, #4840, #10386, #13043, #1864 ) ) ;
#21169=AXIS2_PLACEMENT_3D ( 'NONE', #13699, #5152, #1928 ) ;
#21171=DIRECTION ( 'NONE',  ( 0.000000000000000000, -1.000000000000000000, 0.000000000000000000 ) ) ;
#21176=EDGE_CURVE ( 'NONE', #16109, #14968, #10788, .T. ) ;
#21178=VECTOR ( 'NONE', #1271, 1000.000000000000000 ) ;
#21181=ORIENTED_EDGE ( 'NONE', *, *, #3336, .T. ) ;
#21183=DIRECTION ( 'NONE',  ( -0.000000000000000000, 0.000000000000000000, 1.000000000000000000 ) ) ;
#21195=VECTOR ( 'NONE', #15065, 1000.000000000000000 ) ;
#21199=SHAPE_REPRESENTATION ( 'Heavy Arch Steel Frame Casting', ( #12794 ), #32 ) ;
#21201=EDGE_CURVE ( 'NONE', #19679, #12430, #5230, .T. ) ;
#21204=DIRECTION ( 'NONE',  ( -0.000000000000000000, -0.000000000000000000, 1.000000000000000000 ) ) ;
#21205=EDGE_LOOP ( 'NONE', ( #20996, #3943, #11916, #16751, #13476, #10043 ) ) ;
#21208=ORIENTED_EDGE ( 'NONE', *, *, #2280, .T. ) ;
#21209=ORIENTED_EDGE ( 'NONE', *, *, #11957, .F. ) ;
#21210=CARTESIAN_POINT ( 'NONE',  ( 10.41669750159067220, 217.7548513357008630, -45.00000000000000000 ) ) ;
#21212=LINE ( 'NONE', #14839, #20429 ) ;
#21213=VECTOR ( 'NONE', #5153, 1000.000000000000000 ) ;
#21221=LINE ( 'NONE', #21008, #352 ) ;
#21226=DIRECTION ( 'NONE',  ( 1.000000000000000000, 1.250996701150283068E-16, -0.000000000000000000 ) ) ;
#21227=DIRECTION ( 'NONE',  ( -0.000000000000000000, 0.000000000000000000, 1.000000000000000000 ) ) ;
#21232=ORIENTED_EDGE ( 'NONE', *, *, #8765, .F. ) ;
#21234=ORIENTED_EDGE ( 'NONE', *, *, #14867, .T. ) ;
#21242=LINE ( 'NONE', #14449, #376 ) ;
#21244=CARTESIAN_POINT ( 'NONE',  ( -19.19633154292390032, 45.73157677422673828, 48.68735826550700807 ) ) ;
#21276=DIRECTION ( 'NONE',  ( 0.000000000000000000, 1.000000000000000000, 0.000000000000000000 ) ) ;
#21284=DIRECTION ( 'NONE',  ( 1.000000000000000000, 0.000000000000000000, 0.000000000000000000 ) ) ;
#21293=EDGE_CURVE ( 'NONE', #11997, #2086, #16817, .T. ) ;
#21303=CARTESIAN_POINT ( 'NONE',  ( 116.0391604516428430, 192.9550247130592027, 40.00000000000000000 ) ) ;
#21318=EDGE_CURVE ( 'NONE', #18850, #17724, #2102, .T. ) ;
#21323=DIRECTION ( 'NONE',  ( -1.000000000000000000, 0.000000000000000000, 0.000000000000000000 ) ) ;
#21325=( BOUNDED_CURVE ( )  B_SPLINE_CURVE ( 3, ( #5053, #12164, #18247, #17041 ),
 .UNSPECIFIED., .F., .T. ) 
 B_SPLINE_CURVE_WITH_KNOTS ( ( 4, 4 ),
 ( 3.141592653589793116, 4.712388980384687898 ),
 .UNSPECIFIED. ) 
 CURVE ( )  GEOMETRIC_REPRESENTATION_ITEM ( )  RATIONAL_B_SPLINE_CURVE ( ( 1.000000000000000000, 0.8047378541243654926, 0.8047378541243654926, 1.000000000000000000 ) ) 
 REPRESENTATION_ITEM ( '' )  );
#21329=DIRECTION ( 'NONE',  ( -0.000000000000000000, -0.000000000000000000, 1.000000000000000000 ) ) ;
#21331=AXIS2_PLACEMENT_3D ( 'NONE', #10035, #5065, #8305 ) ;
#21334=ORIENTED_EDGE ( 'NONE', *, *, #10537, .F. ) ;
#21337=EDGE_CURVE ( 'NONE', #12056, #10333, #11931, .T. ) ;
#21338=AXIS2_PLACEMENT_3D ( 'NONE', #13732, #17083, #2158 ) ;
#21351=CARTESIAN_POINT ( 'NONE',  ( -11.50723138933277490, 52.75769294733686365, 46.53163365174636112 ) ) ;
#21362=AXIS2_PLACEMENT_3D ( 'NONE', #11211, #14047, #14265 ) ;
#21363=ORIENTED_EDGE ( 'NONE', *, *, #10887, .T. ) ;
#21364=PLANE ( 'NONE',  #7879 ) ;
#21368=CIRCLE ( 'NONE', #2696, 20.00000000000000000 ) ;
#21370=PLANE ( 'NONE',  #40 ) ;
#21374=CARTESIAN_POINT ( 'NONE',  ( 20.42502041961813930, 230.5765313837437418, -40.00000000000000000 ) ) ;
#21382=VECTOR ( 'NONE', #4376, 1000.000000000000000 ) ;
#21389=CARTESIAN_POINT ( 'NONE',  ( -33.84809828339279392, 56.37865086801084402, -49.33155846391707655 ) ) ;
#21391=EDGE_CURVE ( 'NONE', #20120, #18164, #12107, .T. ) ;
#21408=COLOUR_RGB('Dark Blue',0.08,0.2,0.34);
#21409=FILL_AREA_STYLE_COLOUR('',#21408);
#21410=FILL_AREA_STYLE('',(#21409));
#21411=SURFACE_STYLE_FILL_AREA(#21410);
#21412=SURFACE_SIDE_STYLE('',(#21411));
#21413=SURFACE_STYLE_USAGE(.BOTH.,#21412);
#21414=PRESENTATION_STYLE_ASSIGNMENT((#21413));
ENDSEC;
END-ISO-10303-21;
